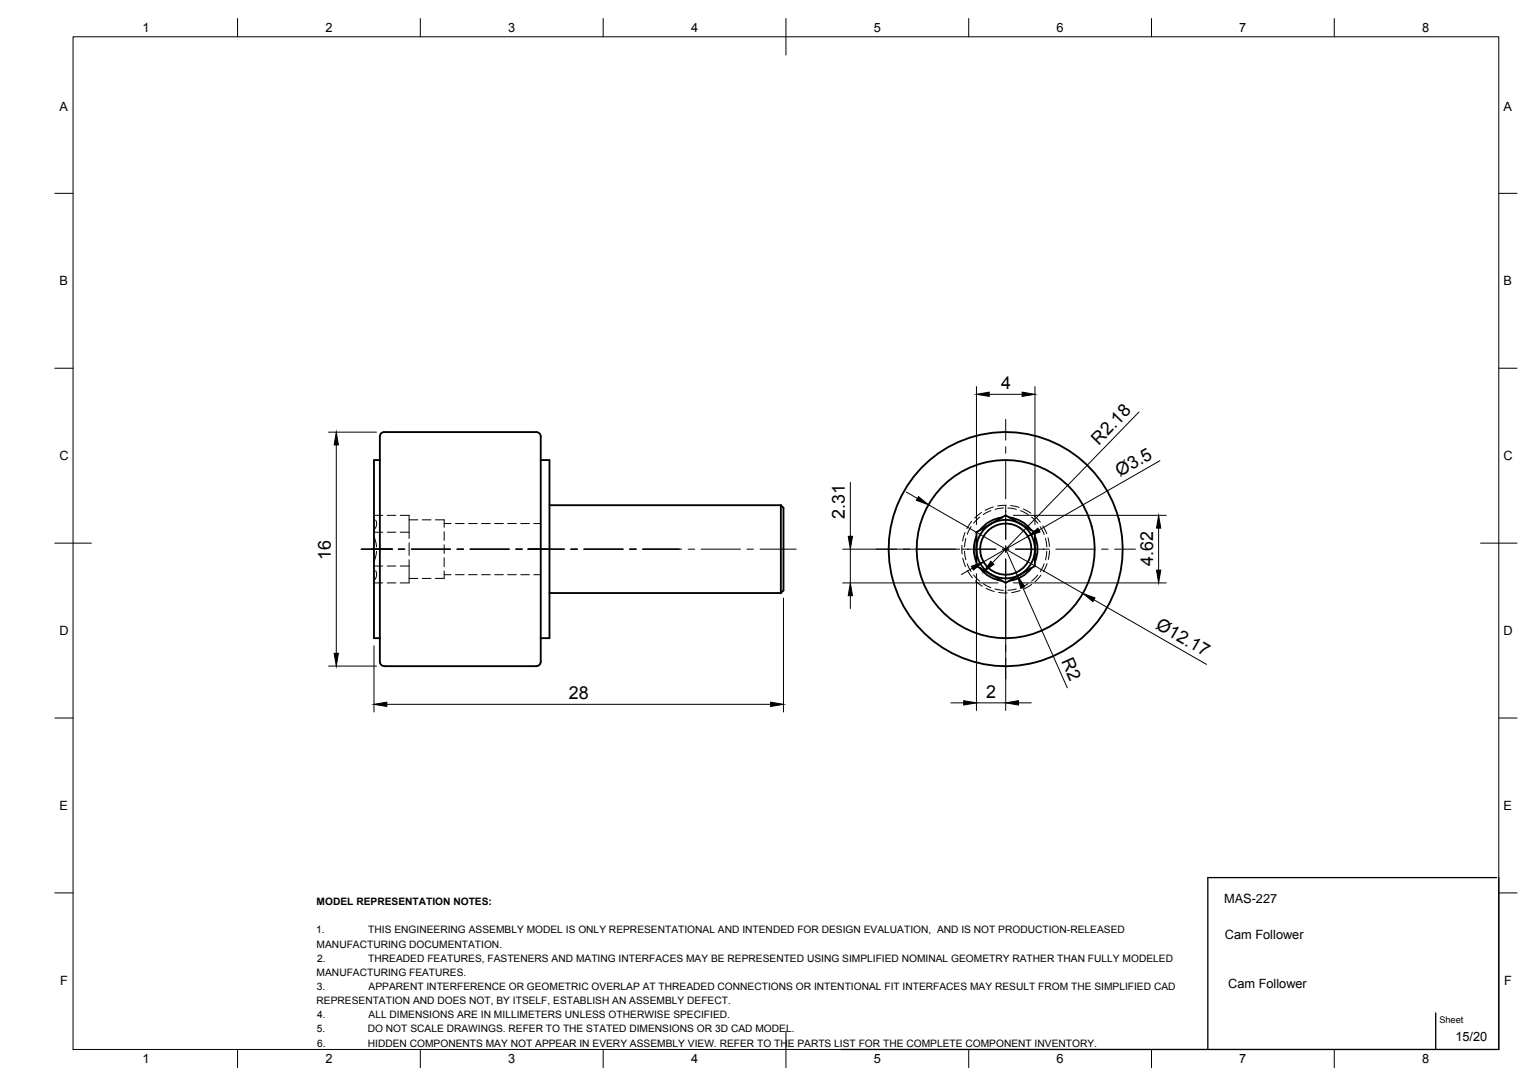
ISO-10303-21;
HEADER;
FILE_DESCRIPTION (('STEP AP214'),
    '1' );
FILE_NAME ( 'Cam Follower.step', '2026-10-06T08:24:41', ( '' ), ( '' ), 'STEP AP214', 'Unspecified', '' );
FILE_SCHEMA (( 'AUTOMOTIVE_DESIGN' ));
ENDSEC;
DATA;
#13=AXIS2_PLACEMENT_3D ( 'NONE', #19056, #4369, #12570 ) ;
#19=( CONVERSION_BASED_UNIT ( 'INCH', #19315 ) LENGTH_UNIT ( ) NAMED_UNIT ( #4330 ) ) ;
#26=AXIS2_PLACEMENT_3D ( 'NONE', #24045, #13033, #11185 ) ;
#76=ORIENTED_EDGE ( 'NONE', *, *, #16694, .F. ) ;
#94=DIRECTION ( 'NONE',  ( -1.000000000000000000, 0.000000000000000000, 0.000000000000000000 ) ) ;
#105=FILL_AREA_STYLE_COLOUR ( '', #1895 ) ;
#111=FACE_OUTER_BOUND ( 'NONE', #23572, .T. ) ;
#122=AXIS2_PLACEMENT_3D ( 'NONE', #22797, #14633, #3420 ) ;
#133=ORIENTED_EDGE ( 'NONE', *, *, #949, .F. ) ;
#142=ORIENTED_EDGE ( 'NONE', *, *, #15280, .T. ) ;
#147=VERTEX_POINT ( 'NONE', #612 ) ;
#148=CARTESIAN_POINT ( 'NONE',  ( 0.07874015748031495954, -0.04546065111729338803, -0.4724409448818898127 ) ) ;
#151=ORIENTED_EDGE ( 'NONE', *, *, #4349, .F. ) ;
#173=FACE_OUTER_BOUND ( 'NONE', #11804, .T. ) ;
#179=VECTOR ( 'NONE', #19878, 39.37007874015748143 ) ;
#197=CARTESIAN_POINT ( 'NONE',  ( -0.3149606299212598381, 0.000000000000000000, -0.03543307086614204404 ) ) ;
#217=CARTESIAN_POINT ( 'NONE',  ( -1.928513779527558736E-17, 0.000000000000000000, -0.4566929133858267376 ) ) ;
#241=EDGE_CURVE ( 'NONE', #21409, #11103, #22772, .T. ) ;
#262=DIRECTION ( 'NONE',  ( 0.8660254037844385966, 0.4999999999999998335, 0.000000000000000000 ) ) ;
#287=LINE ( 'NONE', #8993, #4640 ) ;
#289=ORIENTED_EDGE ( 'NONE', *, *, #13370, .F. ) ;
#294=ORIENTED_EDGE ( 'NONE', *, *, #2324, .F. ) ;
#295=VECTOR ( 'NONE', #17634, 39.37007874015748143 ) ;
#305=VECTOR ( 'NONE', #25355, 39.37007874015748854 ) ;
#307=ORIENTED_EDGE ( 'NONE', *, *, #13471, .F. ) ;
#340=CIRCLE ( 'NONE', #27828, 0.1181102362204724532 ) ;
#402=CYLINDRICAL_SURFACE ( 'NONE', #15048, 0.3149606299212598381 ) ;
#409=AXIS2_PLACEMENT_3D ( 'NONE', #960, #9547, #5473 ) ;
#417=DIRECTION ( 'NONE',  ( -0.000000000000000000, -0.000000000000000000, -1.000000000000000000 ) ) ;
#426=FACE_BOUND ( 'NONE', #2820, .T. ) ;
#444=DIRECTION ( 'NONE',  ( 0.000000000000000000, 0.000000000000000000, 1.000000000000000000 ) ) ;
#511=VECTOR ( 'NONE', #19555, 39.37007874015748143 ) ;
#534=ORIENTED_EDGE ( 'NONE', *, *, #21353, .T. ) ;
#572=CARTESIAN_POINT ( 'NONE',  ( 0.04957542349328453862, 0.06229891813554931657, -0.4653527282821430799 ) ) ;
#597=CARTESIAN_POINT ( 'NONE',  ( -1.928513779527558736E-17, 0.000000000000000000, -0.4448818897637791814 ) ) ;
#612=CARTESIAN_POINT ( 'NONE',  ( 0.07874015748238459567, -0.03414999754297557560, -0.4724409448841456749 ) ) ;
#617=EDGE_CURVE ( 'NONE', #8913, #147, #1095, .T. ) ;
#631=PLANE ( 'NONE',  #22046 ) ;
#638=DIRECTION ( 'NONE',  ( -1.000000000000000000, 0.000000000000000000, 0.000000000000000000 ) ) ;
#647=LINE ( 'NONE', #6869, #25949 ) ;
#681=CARTESIAN_POINT ( 'NONE',  ( 0.07874015748238459567, -0.03414999754297557560, -0.4724409448841456749 ) ) ;
#715=DIRECTION ( 'NONE',  ( 0.4999999999999998890, -0.8660254037844388186, 0.000000000000000000 ) ) ;
#771=AXIS2_PLACEMENT_3D ( 'NONE', #1458, #21348, #1986 ) ;
#785=ORIENTED_EDGE ( 'NONE', *, *, #9722, .F. ) ;
#791=FACE_OUTER_BOUND ( 'NONE', #25595, .T. ) ;
#797=CARTESIAN_POINT ( 'NONE',  ( -1.928513779527558736E-17, 0.000000000000000000, -0.03543307086614204404 ) ) ;
#841=ORIENTED_EDGE ( 'NONE', *, *, #19527, .T. ) ;
#851=AXIS2_PLACEMENT_3D ( 'NONE', #2037, #22857, #17156 ) ;
#859=PLANE ( 'NONE',  #25863 ) ;
#869=CARTESIAN_POINT ( 'NONE',  ( 0.06889763779527550980, 8.437527159479786693E-18, -0.2834645669291338543 ) ) ;
#876=DIRECTION ( 'NONE',  ( -0.8660254037844388186, 0.4999999999999998890, 0.000000000000000000 ) ) ;
#889=CIRCLE ( 'NONE', #13953, 0.08582677165167480748 ) ;
#895=FACE_OUTER_BOUND ( 'NONE', #5397, .T. ) ;
#922=ADVANCED_BREP_SHAPE_REPRESENTATION ( 'Cam Follower', ( #12666, #11588 ), #22004 ) ;
#926=SHAPE_DEFINITION_REPRESENTATION ( #15254, #6338 ) ;
#947=DIRECTION ( 'NONE',  ( 0.000000000000000000, 1.000000000000000000, 0.000000000000000000 ) ) ;
#949=EDGE_CURVE ( 'NONE', #26096, #20147, #2007, .T. ) ;
#960=CARTESIAN_POINT ( 'NONE',  ( -1.466875984251968630E-17, 0.000000000000000000, 0.000000000000000000 ) ) ;
#992=EDGE_CURVE ( 'NONE', #13219, #8587, #11932, .T. ) ;
#1028=DIRECTION ( 'NONE',  ( 0.000000000000000000, 0.000000000000000000, -1.000000000000000000 ) ) ;
#1072=AXIS2_PLACEMENT_3D ( 'NONE', #797, #26485, #22259 ) ;
#1076=ORIENTED_EDGE ( 'NONE', *, *, #5071, .F. ) ;
#1095=CIRCLE ( 'NONE', #20479, 0.08582677165167480748 ) ;
#1109=EDGE_CURVE ( 'NONE', #8913, #147, #3613, .T. ) ;
#1139=DIRECTION ( 'NONE',  ( 0.000000000000000000, 0.000000000000000000, 1.000000000000000000 ) ) ;
#1154=APPLICATION_CONTEXT ( 'automotive_design' ) ;
#1176=CARTESIAN_POINT ( 'NONE',  ( -0.009795313329799356164, 0.08526597544922019656, -0.4724409448841456749 ) ) ;
#1190=CARTESIAN_POINT ( 'NONE',  ( -0.08582677165167483524, 0.000000000000000000, -0.4724409448818898127 ) ) ;
#1215=ADVANCED_FACE ( 'NONE', ( #11828 ), #5648, .F. ) ;
#1220=LINE ( 'NONE', #9824, #25523 ) ;
#1227=DIRECTION ( 'NONE',  ( 1.000000000000000000, 0.000000000000000000, 0.000000000000000000 ) ) ;
#1268=DIRECTION ( 'NONE',  ( 0.000000000000000000, -1.000000000000000000, 0.000000000000000000 ) ) ;
#1279=DIRECTION ( 'NONE',  ( 1.000000000000000000, 0.000000000000000000, -0.000000000000000000 ) ) ;
#1309=DIRECTION ( 'NONE',  ( -1.000000000000000000, 0.000000000000000000, 0.000000000000000000 ) ) ;
#1314=AXIS2_PLACEMENT_3D ( 'NONE', #18114, #26761, #16038 ) ;
#1339=ORIENTED_EDGE ( 'NONE', *, *, #16589, .T. ) ;
#1349=CARTESIAN_POINT ( 'NONE',  ( 0.009795313329541911057, 0.08526597544697904485, -0.4724409448818898127 ) ) ;
#1370=DIRECTION ( 'NONE',  ( -0.000000000000000000, -0.000000000000000000, -1.000000000000000000 ) ) ;
#1407=ADVANCED_FACE ( 'NONE', ( #8707 ), #25945, .T. ) ;
#1444=EDGE_CURVE ( 'NONE', #22435, #24921, #647, .T. ) ;
#1458=CARTESIAN_POINT ( 'NONE',  ( -0.3031496062992123375, 0.000000000000000000, -0.03543307086614204404 ) ) ;
#1463=ORIENTED_EDGE ( 'NONE', *, *, #27662, .F. ) ;
#1464=CIRCLE ( 'NONE', #9132, 0.07874015748031489015 ) ;
#1465=DIRECTION ( 'NONE',  ( 0.000000000000000000, 0.000000000000000000, 1.000000000000000000 ) ) ;
#1467=AXIS2_PLACEMENT_3D ( 'NONE', #24695, #4934, #13548 ) ;
#1502=EDGE_CURVE ( 'NONE', #20698, #22435, #15499, .T. ) ;
#1510=FACE_OUTER_BOUND ( 'NONE', #14210, .T. ) ;
#1543=DIRECTION ( 'NONE',  ( 0.000000000000000000, 0.000000000000000000, -1.000000000000000000 ) ) ;
#1557=EDGE_LOOP ( 'NONE', ( #14465, #20326, #18276, #7986 ) ) ;
#1673=VERTEX_POINT ( 'NONE', #23799 ) ;
#1675=DIRECTION ( 'NONE',  ( -0.000000000000000000, -0.000000000000000000, -1.000000000000000000 ) ) ;
#1685=EDGE_CURVE ( 'NONE', #20128, #15627, #22080, .T. ) ;
#1708=EDGE_CURVE ( 'NONE', #2756, #15627, #3356, .T. ) ;
#1714=CIRCLE ( 'NONE', #26498, 0.2395669291338582696 ) ;
#1770=ORIENTED_EDGE ( 'NONE', *, *, #6491, .F. ) ;
#1867=VERTEX_POINT ( 'NONE', #26724 ) ;
#1873=CYLINDRICAL_SURFACE ( 'NONE', #17851, 0.2395669291338582696 ) ;
#1884=CARTESIAN_POINT ( 'NONE',  ( 0.07874015748031489015, 9.642888182262615344E-18, -0.3779527559055118058 ) ) ;
#1891=FACE_OUTER_BOUND ( 'NONE', #4069, .T. ) ;
#1895=COLOUR_RGB ( '', 0.40784314, 0.44705882, 0.49803922) ;
#1934=VERTEX_POINT ( 'NONE', #24403 ) ;
#1956=AXIS2_PLACEMENT_3D ( 'NONE', #9250, #22687, #14227 ) ;
#1962=ORIENTED_EDGE ( 'NONE', *, *, #1502, .T. ) ;
#1965=CARTESIAN_POINT ( 'NONE',  ( -1.928513779527558736E-17, 0.000000000000000000, -0.4566929133858267376 ) ) ;
#1986=DIRECTION ( 'NONE',  ( 0.000000000000000000, 0.000000000000000000, -1.000000000000000000 ) ) ;
#2007=CIRCLE ( 'NONE', #5137, 0.3149606299212598381 ) ;
#2037=CARTESIAN_POINT ( 'NONE',  ( 0.3031496062992122820, 3.712511950171106268E-17, -0.4448818897637791814 ) ) ;
#2066=EDGE_CURVE ( 'NONE', #2885, #6378, #9145, .T. ) ;
#2067=AXIS2_PLACEMENT_3D ( 'NONE', #10228, #4171, #8271 ) ;
#2129=ORIENTED_EDGE ( 'NONE', *, *, #13165, .F. ) ;
#2130=DIRECTION ( 'NONE',  ( 0.000000000000000000, 0.000000000000000000, -1.000000000000000000 ) ) ;
#2139=DIRECTION ( 'NONE',  ( -0.000000000000000000, -0.000000000000000000, -1.000000000000000000 ) ) ;
#2160=FACE_OUTER_BOUND ( 'NONE', #7511, .T. ) ;
#2171=CARTESIAN_POINT ( 'NONE',  ( 0.06894484415258525511, 0.05111597790624471116, -0.4724409448841456749 ) ) ;
#2198=LINE ( 'NONE', #2975, #8961 ) ;
#2218=ORIENTED_EDGE ( 'NONE', *, *, #241, .T. ) ;
#2227=ORIENTED_EDGE ( 'NONE', *, *, #22042, .F. ) ;
#2247=VERTEX_POINT ( 'NONE', #1349 ) ;
#2259=CARTESIAN_POINT ( 'NONE',  ( 0.000000000000000000, 0.000000000000000000, -0.4724409448818898127 ) ) ;
#2305=DIRECTION ( 'NONE',  ( -1.000000000000000000, 0.000000000000000000, 0.000000000000000000 ) ) ;
#2324=EDGE_CURVE ( 'NONE', #1867, #20809, #4761, .T. ) ;
#2360=EDGE_CURVE ( 'NONE', #24921, #21448, #25528, .T. ) ;
#2372=EDGE_CURVE ( 'NONE', #7271, #14162, #6429, .T. ) ;
#2381=ADVANCED_FACE ( 'NONE', ( #111 ), #4035, .F. ) ;
#2387=DIRECTION ( 'NONE',  ( 0.8660254037844382635, 0.5000000000000005551, 0.000000000000000000 ) ) ;
#2407=EDGE_LOOP ( 'NONE', ( #13278, #3298, #13573, #24116, #10984, #25647 ) ) ;
#2436=AXIS2_PLACEMENT_3D ( 'NONE', #217, #23645, #21376 ) ;
#2447=FILL_AREA_STYLE ('',( #105 ) ) ;
#2457=ORIENTED_EDGE ( 'NONE', *, *, #2066, .T. ) ;
#2463=FACE_OUTER_BOUND ( 'NONE', #1557, .T. ) ;
#2466=EDGE_CURVE ( 'NONE', #21409, #9119, #2876, .T. ) ;
#2467=PLANE ( 'NONE',  #7333 ) ;
#2492=DIRECTION ( 'NONE',  ( -1.000000000000000000, 0.000000000000000000, 0.000000000000000000 ) ) ;
#2513=LINE ( 'NONE', #7039, #22957 ) ;
#2525=CYLINDRICAL_SURFACE ( 'NONE', #25674, 0.1181102362204724532 ) ;
#2547=PLANE ( 'NONE',  #12830 ) ;
#2570=EDGE_CURVE ( 'NONE', #12477, #20698, #19211, .T. ) ;
#2582=LINE ( 'NONE', #17062, #18450 ) ;
#2590=DIRECTION ( 'NONE',  ( 1.000000000000000000, 0.000000000000000000, 0.000000000000000000 ) ) ;
#2632=AXIS2_PLACEMENT_3D ( 'NONE', #14783, #10215, #18829 ) ;
#2639=AXIS2_PLACEMENT_3D ( 'NONE', #27845, #16966, #4383 ) ;
#2650=CYLINDRICAL_SURFACE ( 'NONE', #4021, 0.3149606299212598381 ) ;
#2653=DIRECTION ( 'NONE',  ( -0.000000000000000000, -0.000000000000000000, -1.000000000000000000 ) ) ;
#2686=CIRCLE ( 'NONE', #13519, 0.07874015748031489015 ) ;
#2695=AXIS2_PLACEMENT_3D ( 'NONE', #25972, #417, #8999 ) ;
#2721=ORIENTED_EDGE ( 'NONE', *, *, #27018, .T. ) ;
#2732=DIRECTION ( 'NONE',  ( 0.000000000000000000, 0.000000000000000000, -1.000000000000000000 ) ) ;
#2744=CARTESIAN_POINT ( 'NONE',  ( 0.000000000000000000, 0.000000000000000000, -0.4724409448841456749 ) ) ;
#2756=VERTEX_POINT ( 'NONE', #6727 ) ;
#2768=EDGE_CURVE ( 'NONE', #7482, #18177, #8831, .T. ) ;
#2799=AXIS2_PLACEMENT_3D ( 'NONE', #20368, #22920, #1028 ) ;
#2820=EDGE_LOOP ( 'NONE', ( #12186, #18779 ) ) ;
#2876=B_SPLINE_CURVE_WITH_KNOTS ( 'NONE', 3,
 ( #15346, #23939, #8947, #6846, #15472, #15608 ),
 .UNSPECIFIED., .F., .F.,
 ( 4, 2, 4 ),
 ( 0.002631077521236949331, 0.003072896085239190580, 0.003514714649241431829 ),
 .UNSPECIFIED. ) ;
#2885=VERTEX_POINT ( 'NONE', #24357 ) ;
#2909=EDGE_CURVE ( 'NONE', #4618, #17370, #9814, .T. ) ;
#2928=ORIENTED_EDGE ( 'NONE', *, *, #27409, .F. ) ;
#2944=CARTESIAN_POINT ( 'NONE',  ( 0.01453548245982153216, 0.08252923752360777354, -0.4702630791244896136 ) ) ;
#2975=CARTESIAN_POINT ( 'NONE',  ( 0.06894484415506239861, -0.05111597790242464190, -0.4724409448818898127 ) ) ;
#2997=CARTESIAN_POINT ( 'NONE',  ( -0.06894484415077309358, 0.05111597790490104293, -0.4724409448818898127 ) ) ;
#3044=FACE_OUTER_BOUND ( 'NONE', #26076, .T. ) ;
#3065=AXIS2_PLACEMENT_3D ( 'NONE', #13857, #11454, #876 ) ;
#3066=ORIENTED_EDGE ( 'NONE', *, *, #5730, .T. ) ;
#3096=ORIENTED_EDGE ( 'NONE', *, *, #1444, .F. ) ;
#3114=ORIENTED_EDGE ( 'NONE', *, *, #27574, .T. ) ;
#3126=CARTESIAN_POINT ( 'NONE',  ( -4.821283464566928349E-18, 0.000000000000000000, -0.2834645669291338543 ) ) ;
#3238=DIRECTION ( 'NONE',  ( -0.000000000000000000, -0.000000000000000000, -1.000000000000000000 ) ) ;
#3242=CARTESIAN_POINT ( 'NONE',  ( -0.2395669291338582696, 0.000000000000000000, -0.4724409448818898127 ) ) ;
#3259=CARTESIAN_POINT ( 'NONE',  ( -0.06894484415077309358, 0.05111597790490104293, -0.4724409448818898127 ) ) ;
#3298=ORIENTED_EDGE ( 'NONE', *, *, #16372, .F. ) ;
#3301=FACE_OUTER_BOUND ( 'NONE', #4635, .T. ) ;
#3318=CARTESIAN_POINT ( 'NONE',  ( 0.2395669291338582696, 2.933848729453403498E-17, 0.000000000000000000 ) ) ;
#3329=EDGE_CURVE ( 'NONE', #8587, #13219, #1714, .T. ) ;
#3342=ORIENTED_EDGE ( 'NONE', *, *, #949, .T. ) ;
#3356=CIRCLE ( 'NONE', #21900, 0.07874015748031489015 ) ;
#3420=DIRECTION ( 'NONE',  ( -1.000000000000000000, 0.000000000000000000, 0.000000000000000000 ) ) ;
#3442=CARTESIAN_POINT ( 'NONE',  ( -0.07874015748031489015, 0.000000000000000000, -0.3779527559055118058 ) ) ;
#3527=CIRCLE ( 'NONE', #12131, 0.07874015748031489015 ) ;
#3542=VERTEX_POINT ( 'NONE', #27613 ) ;
#3573=ADVANCED_FACE ( 'NONE', ( #1891 ), #18981, .F. ) ;
#3579=VERTEX_POINT ( 'NONE', #17015 ) ;
#3597=ORIENTED_EDGE ( 'NONE', *, *, #10686, .F. ) ;
#3613=B_SPLINE_CURVE_WITH_KNOTS ( 'NONE', 3,
 ( #11138, #9009, #19895, #17630, #26250, #6910, #20029, #681 ),
 .UNSPECIFIED., .F., .F.,
 ( 4, 2, 2, 4 ),
 ( 0.001552469560294957029, 0.001994063167382608553, 0.002435656774470260078, 0.003318843988645562692 ),
 .UNSPECIFIED. ) ;
#3622=DIRECTION ( 'NONE',  ( 0.000000000000000000, 0.000000000000000000, -1.000000000000000000 ) ) ;
#3630=VERTEX_POINT ( 'NONE', #2171 ) ;
#3645=CARTESIAN_POINT ( 'NONE',  ( 0.000000000000000000, 0.000000000000000000, -0.4724409448841456749 ) ) ;
#3654=EDGE_CURVE ( 'NONE', #1673, #2756, #24054, .T. ) ;
#3665=DIRECTION ( 'NONE',  ( 0.000000000000000000, 0.000000000000000000, 1.000000000000000000 ) ) ;
#3684=PLANE ( 'NONE',  #4186 ) ;
#3699=ORIENTED_EDGE ( 'NONE', *, *, #19527, .F. ) ;
#3739=ORIENTED_EDGE ( 'NONE', *, *, #25748, .T. ) ;
#3769=AXIS2_PLACEMENT_3D ( 'NONE', #26947, #26798, #11404 ) ;
#3803=ADVANCED_FACE ( 'NONE', ( #1510 ), #25378, .F. ) ;
#3834=DIRECTION ( 'NONE',  ( -1.000000000000000000, -1.224646799147353454E-16, 0.000000000000000000 ) ) ;
#3868=VERTEX_POINT ( 'NONE', #7738 ) ;
#3871=CARTESIAN_POINT ( 'NONE',  ( -0.1110236220424516002, 0.000000000000000000, 0.6299212598425196763 ) ) ;
#3898=DIRECTION ( 'NONE',  ( 1.000000000000000000, 0.000000000000000000, 0.000000000000000000 ) ) ;
#3907=DIRECTION ( 'NONE',  ( 0.000000000000000000, 0.000000000000000000, 1.000000000000000000 ) ) ;
#3913=EDGE_LOOP ( 'NONE', ( #12682, #15515, #133, #1463 ) ) ;
#3963=DIRECTION ( 'NONE',  ( -0.000000000000000000, -0.000000000000000000, -1.000000000000000000 ) ) ;
#3986=CARTESIAN_POINT ( 'NONE',  ( 0.01928643301569668220, -0.07978627494126659669, -0.4680802598521938696 ) ) ;
#3995=EDGE_CURVE ( 'NONE', #26096, #10570, #24430, .T. ) ;
#4021=AXIS2_PLACEMENT_3D ( 'NONE', #24533, #11277, #15663 ) ;
#4035=PLANE ( 'NONE',  #25072 ) ;
#4061=VECTOR ( 'NONE', #262, 39.37007874015748854 ) ;
#4069=EDGE_LOOP ( 'NONE', ( #3739, #21924, #24634, #76, #3096, #7987, #5002 ) ) ;
#4091=CARTESIAN_POINT ( 'NONE',  ( 0.3031496062992122820, 3.784833611538078052E-17, -0.4566929133858267376 ) ) ;
#4123=EDGE_LOOP ( 'NONE', ( #4562, #26365 ) ) ;
#4170=EDGE_LOOP ( 'NONE', ( #7045, #1962, #27253 ) ) ;
#4171=DIRECTION ( 'NONE',  ( 0.000000000000000000, 0.000000000000000000, 1.000000000000000000 ) ) ;
#4172=CARTESIAN_POINT ( 'NONE',  ( 0.1110236220424516002, 1.359647233640338808E-17, 0.6299212598425196763 ) ) ;
#4186=AXIS2_PLACEMENT_3D ( 'NONE', #19375, #25313, #16985 ) ;
#4207=EDGE_LOOP ( 'NONE', ( #15106, #13124 ) ) ;
#4221=EDGE_LOOP ( 'NONE', ( #24244, #2218, #3066 ) ) ;
#4238=DIRECTION ( 'NONE',  ( -1.000000000000000000, 0.000000000000000000, 0.000000000000000000 ) ) ;
#4239=CARTESIAN_POINT ( 'NONE',  ( 0.000000000000000000, 0.000000000000000000, -0.4724409448818898127 ) ) ;
#4297=PRODUCT_DEFINITION_CONTEXT ( 'detailed design', #1154, 'design' ) ;
#4316=DIRECTION ( 'NONE',  ( 0.000000000000000000, 0.000000000000000000, -1.000000000000000000 ) ) ;
#4330=DIMENSIONAL_EXPONENTS ( 1.000000000000000000, 0.000000000000000000, 0.000000000000000000, 0.000000000000000000, 0.000000000000000000, 0.000000000000000000, 0.000000000000000000 ) ;
#4346=ORIENTED_EDGE ( 'NONE', *, *, #2909, .T. ) ;
#4349=EDGE_CURVE ( 'NONE', #7482, #3868, #8097, .T. ) ;
#4353=TOROIDAL_SURFACE ( 'NONE', #21954, 0.3031496062992122820, 0.01181102362204755792 ) ;
#4369=DIRECTION ( 'NONE',  ( 0.000000000000000000, 0.000000000000000000, -1.000000000000000000 ) ) ;
#4383=DIRECTION ( 'NONE',  ( -1.000000000000000000, 0.000000000000000000, 0.000000000000000000 ) ) ;
#4493=DIRECTION ( 'NONE',  ( -0.000000000000000000, -0.000000000000000000, -1.000000000000000000 ) ) ;
#4506=EDGE_CURVE ( 'NONE', #12477, #26781, #2582, .T. ) ;
#4562=ORIENTED_EDGE ( 'NONE', *, *, #2324, .T. ) ;
#4611=VECTOR ( 'NONE', #3907, 39.37007874015748143 ) ;
#4614=FACE_OUTER_BOUND ( 'NONE', #15635, .T. ) ;
#4618=VERTEX_POINT ( 'NONE', #22357 ) ;
#4623=CARTESIAN_POINT ( 'NONE',  ( -0.07874015748031495954, -0.04546065111729338803, -0.4724409448818898127 ) ) ;
#4635=EDGE_LOOP ( 'NONE', ( #142, #12752 ) ) ;
#4640=VECTOR ( 'NONE', #11392, 39.37007874015748143 ) ;
#4679=EDGE_CURVE ( 'NONE', #14162, #3630, #27583, .T. ) ;
#4687=CARTESIAN_POINT ( 'NONE',  ( 0.000000000000000000, 0.000000000000000000, -0.4724409448841456749 ) ) ;
#4690=DIRECTION ( 'NONE',  ( -0.8660254037844382635, -0.5000000000000005551, 0.000000000000000000 ) ) ;
#4727=EDGE_LOOP ( 'NONE', ( #14075, #24927 ) ) ;
#4742=LINE ( 'NONE', #148, #10499 ) ;
#4761=CIRCLE ( 'NONE', #2067, 0.1110236220424516002 ) ;
#4767=FACE_OUTER_BOUND ( 'NONE', #8375, .T. ) ;
#4805=VERTEX_POINT ( 'NONE', #21773 ) ;
#4825=CARTESIAN_POINT ( 'NONE',  ( 0.07874015748031495954, 0.04546065111729338803, -0.3779527559055118058 ) ) ;
#4834=FACE_BOUND ( 'NONE', #5849, .T. ) ;
#4835=ADVANCED_FACE ( 'NONE', ( #3044 ), #5041, .T. ) ;
#4860=CARTESIAN_POINT ( 'NONE',  ( -1.466875984251968630E-17, 0.000000000000000000, -0.4724409448818898127 ) ) ;
#4884=FACE_OUTER_BOUND ( 'NONE', #19252, .T. ) ;
#4934=DIRECTION ( 'NONE',  ( 0.000000000000000000, 0.000000000000000000, -1.000000000000000000 ) ) ;
#4935=ORIENTED_EDGE ( 'NONE', *, *, #25296, .T. ) ;
#4949=ORIENTED_EDGE ( 'NONE', *, *, #11130, .F. ) ;
#4950=DIRECTION ( 'NONE',  ( 0.000000000000000000, -1.000000000000000000, 0.000000000000000000 ) ) ;
#4962=DIRECTION ( 'NONE',  ( -1.000000000000000000, 0.000000000000000000, 0.000000000000000000 ) ) ;
#4991=DIRECTION ( 'NONE',  ( 0.000000000000000000, -1.000000000000000000, 0.000000000000000000 ) ) ;
#5002=ORIENTED_EDGE ( 'NONE', *, *, #16148, .F. ) ;
#5010=DIRECTION ( 'NONE',  ( -1.000000000000000000, 0.000000000000000000, 0.000000000000000000 ) ) ;
#5041=CYLINDRICAL_SURFACE ( 'NONE', #409, 0.2395669291338582696 ) ;
#5045=CARTESIAN_POINT ( 'NONE',  ( -0.05945372446461825305, -0.05659567841061365762, -0.4680802598521939806 ) ) ;
#5054=FACE_OUTER_BOUND ( 'NONE', #11043, .T. ) ;
#5071=EDGE_CURVE ( 'NONE', #26781, #27801, #26866, .T. ) ;
#5080=DIRECTION ( 'NONE',  ( 0.000000000000000000, 0.000000000000000000, -1.000000000000000000 ) ) ;
#5083=ORIENTED_EDGE ( 'NONE', *, *, #19523, .F. ) ;
#5089=ORIENTED_EDGE ( 'NONE', *, *, #18442, .T. ) ;
#5121=CARTESIAN_POINT ( 'NONE',  ( -1.466875984251968630E-17, 0.000000000000000000, -0.02362204724409448786 ) ) ;
#5123=DIRECTION ( 'NONE',  ( -1.000000000000000000, 0.000000000000000000, 0.000000000000000000 ) ) ;
#5124=ORIENTED_EDGE ( 'NONE', *, *, #22846, .T. ) ;
#5125=AXIS2_PLACEMENT_3D ( 'NONE', #13732, #11340, #15599 ) ;
#5130=VECTOR ( 'NONE', #4991, 39.37007874015748143 ) ;
#5137=AXIS2_PLACEMENT_3D ( 'NONE', #27832, #8468, #4238 ) ;
#5183=CARTESIAN_POINT ( 'NONE',  ( -0.009795313329541911057, -0.08526597544697904485, -0.4724409448818898127 ) ) ;
#5212=CARTESIAN_POINT ( 'NONE',  ( 0.2395669291338582696, 2.933848729453403498E-17, -0.4566929133858267376 ) ) ;
#5213=CARTESIAN_POINT ( 'NONE',  ( 0.05945372446461825305, 0.05659567841061365762, -0.4680802598521939806 ) ) ;
#5229=CARTESIAN_POINT ( 'NONE',  ( 0.000000000000000000, 0.000000000000000000, 0.000000000000000000 ) ) ;
#5267=VERTEX_POINT ( 'NONE', #9743 ) ;
#5273=ORIENTED_EDGE ( 'NONE', *, *, #11599, .T. ) ;
#5294=VECTOR ( 'NONE', #1675, 39.37007874015748143 ) ;
#5312=VERTEX_POINT ( 'NONE', #23330 ) ;
#5315=LINE ( 'NONE', #20291, #27238 ) ;
#5357=ADVANCED_FACE ( 'NONE', ( #4767 ), #2650, .T. ) ;
#5361=LINE ( 'NONE', #5212, #18750 ) ;
#5363=CIRCLE ( 'NONE', #851, 0.01181102362204754924 ) ;
#5397=EDGE_LOOP ( 'NONE', ( #10780, #27110 ) ) ;
#5424=EDGE_CURVE ( 'NONE', #20128, #6015, #2513, .T. ) ;
#5430=ORIENTED_EDGE ( 'NONE', *, *, #2909, .F. ) ;
#5441=UNCERTAINTY_MEASURE_WITH_UNIT (LENGTH_MEASURE( 1.000000000000000082E-05 ), #19, 'distance_accuracy_value', 'NONE') ;
#5472=EDGE_CURVE ( 'NONE', #10266, #9518, #21080, .T. ) ;
#5473=DIRECTION ( 'NONE',  ( -1.000000000000000000, 0.000000000000000000, 0.000000000000000000 ) ) ;
#5499=MECHANICAL_DESIGN_GEOMETRIC_PRESENTATION_REPRESENTATION('',(#27617),#17674);
#5507=DIRECTION ( 'NONE',  ( -1.000000000000000000, 0.000000000000000000, 0.000000000000000000 ) ) ;
#5517=CARTESIAN_POINT ( 'NONE',  ( -9.160727710493059047E-17, 0.000000000000000000, -0.02362204724409468909 ) ) ;
#5543=CARTESIAN_POINT ( 'NONE',  ( -0.08582677165393072516, 0.000000000000000000, -0.4724409448841456749 ) ) ;
#5552=EDGE_CURVE ( 'NONE', #23745, #23749, #5363, .T. ) ;
#5586=ADVANCED_FACE ( 'NONE', ( #18590 ), #13959, .T. ) ;
#5589=LINE ( 'NONE', #3442, #7088 ) ;
#5615=ORIENTED_EDGE ( 'NONE', *, *, #7592, .T. ) ;
#5635=VERTEX_POINT ( 'NONE', #7883 ) ;
#5648=CONICAL_SURFACE ( 'NONE', #25034, 0.08582677165393072516, 0.7853981625000011624 ) ;
#5661=ORIENTED_EDGE ( 'NONE', *, *, #13984, .T. ) ;
#5689=AXIS2_PLACEMENT_3D ( 'NONE', #21404, #8545, #17163 ) ;
#5730=EDGE_CURVE ( 'NONE', #11103, #9119, #22977, .T. ) ;
#5738=ADVANCED_FACE ( 'NONE', ( #8467 ), #22051, .F. ) ;
#5770=DIRECTION ( 'NONE',  ( 0.000000000000000000, 0.000000000000000000, -1.000000000000000000 ) ) ;
#5834=CARTESIAN_POINT ( 'NONE',  ( 0.04448665381632212201, -0.06523692067838748887, -0.4653551329966303385 ) ) ;
#5849=EDGE_LOOP ( 'NONE', ( #7073, #17608 ) ) ;
#5881=EDGE_CURVE ( 'NONE', #2885, #8441, #18904, .T. ) ;
#5915=ORIENTED_EDGE ( 'NONE', *, *, #27409, .T. ) ;
#6015=VERTEX_POINT ( 'NONE', #17564 ) ;
#6024=AXIS2_PLACEMENT_3D ( 'NONE', #19196, #23324, #18909 ) ;
#6030=EDGE_LOOP ( 'NONE', ( #3114, #9421 ) ) ;
#6058=ORIENTED_EDGE ( 'NONE', *, *, #7177, .T. ) ;
#6116=ORIENTED_EDGE ( 'NONE', *, *, #617, .T. ) ;
#6120=CARTESIAN_POINT ( 'NONE',  ( 0.06894484415077314909, -0.05111597790490109150, -0.4724409448818898127 ) ) ;
#6135=DIRECTION ( 'NONE',  ( -1.000000000000000000, 0.000000000000000000, 0.000000000000000000 ) ) ;
#6161=ORIENTED_EDGE ( 'NONE', *, *, #1708, .F. ) ;
#6174=ORIENTED_EDGE ( 'NONE', *, *, #23058, .F. ) ;
#6194=CARTESIAN_POINT ( 'NONE',  ( 0.000000000000000000, 0.000000000000000000, -0.3779527559055118058 ) ) ;
#6252=CARTESIAN_POINT ( 'NONE',  ( -4.821283464566928349E-18, 0.000000000000000000, -0.3779527559055118058 ) ) ;
#6277=LINE ( 'NONE', #3871, #10048 ) ;
#6285=VECTOR ( 'NONE', #11721, 39.37007874015748143 ) ;
#6302=AXIS2_PLACEMENT_3D ( 'NONE', #12976, #17365, #8604 ) ;
#6308=ORIENTED_EDGE ( 'NONE', *, *, #23058, .T. ) ;
#6338=SHAPE_REPRESENTATION ( 'Cam Follower', ( #11588 ), #22004 ) ;
#6340=ADVANCED_FACE ( 'NONE', ( #11819 ), #20435, .F. ) ;
#6378=VERTEX_POINT ( 'NONE', #16763 ) ;
#6429=LINE ( 'NONE', #18844, #27794 ) ;
#6467=CARTESIAN_POINT ( 'NONE',  ( 0.000000000000000000, 0.000000000000000000, 0.6299212598425196763 ) ) ;
#6475=CARTESIAN_POINT ( 'NONE',  ( -1.928513779527558736E-17, 0.000000000000000000, -0.4448818897637791814 ) ) ;
#6488=CARTESIAN_POINT ( 'NONE',  ( -0.07874015748031495954, -1.062017969535966354E-23, -0.4653543306978102367 ) ) ;
#6491=EDGE_CURVE ( 'NONE', #6015, #5312, #26470, .T. ) ;
#6500=LINE ( 'NONE', #27562, #14787 ) ;
#6532=ORIENTED_EDGE ( 'NONE', *, *, #24900, .T. ) ;
#6566=SURFACE_STYLE_FILL_AREA ( #2447 ) ;
#6635=CARTESIAN_POINT ( 'NONE',  ( 0.07874015748031495954, 0.04546065111729338803, -0.4724409448818898127 ) ) ;
#6672=ORIENTED_EDGE ( 'NONE', *, *, #14295, .T. ) ;
#6678=CARTESIAN_POINT ( 'NONE',  ( 0.000000000000000000, -0.09092130223458683158, -0.3779527559055118058 ) ) ;
#6723=AXIS2_PLACEMENT_3D ( 'NONE', #14094, #5770, #14250 ) ;
#6724=CARTESIAN_POINT ( 'NONE',  ( 0.000000000000000000, 0.000000000000000000, -0.4724409448818898127 ) ) ;
#6727=CARTESIAN_POINT ( 'NONE',  ( 0.03937007874015749365, -0.06819097667593998491, -0.3779527559055118058 ) ) ;
#6766=AXIS2_PLACEMENT_3D ( 'NONE', #7584, #14084, #22698 ) ;
#6829=ORIENTED_EDGE ( 'NONE', *, *, #20642, .T. ) ;
#6841=CARTESIAN_POINT ( 'NONE',  ( 0.000000000000000000, -0.09092130223458683158, -0.3779527559055118058 ) ) ;
#6846=CARTESIAN_POINT ( 'NONE',  ( -0.07874015748031495954, 0.02307066120096010892, -0.4684762439721033012 ) ) ;
#6869=CARTESIAN_POINT ( 'NONE',  ( 0.000000000000000000, 0.09092130223458683158, -0.3779527559055118058 ) ) ;
#6871=CARTESIAN_POINT ( 'NONE',  ( -0.03937007874015754916, -0.06819097667594005430, -0.3779527559055118058 ) ) ;
#6876=EDGE_LOOP ( 'NONE', ( #6058, #6672 ) ) ;
#6877=AXIS2_PLACEMENT_3D ( 'NONE', #16800, #7907, #20474 ) ;
#6909=CARTESIAN_POINT ( 'NONE',  ( -0.06894484415258525511, -0.05111597790624471116, -0.4724409448841456749 ) ) ;
#6910=CARTESIAN_POINT ( 'NONE',  ( 0.07874015748031498729, -0.01181388133159171419, -0.4653549736499515421 ) ) ;
#6941=CARTESIAN_POINT ( 'NONE',  ( 0.000000000000000000, 0.000000000000000000, 0.6299212598425196763 ) ) ;
#6984=AXIS2_PLACEMENT_3D ( 'NONE', #26690, #22465, #18627 ) ;
#7026=ORIENTED_EDGE ( 'NONE', *, *, #16884, .T. ) ;
#7039=CARTESIAN_POINT ( 'NONE',  ( 0.000000000000000000, -0.09092130223458683158, -0.3779527559055118058 ) ) ;
#7042=CARTESIAN_POINT ( 'NONE',  ( 0.06889763779527550980, 0.000000000000000000, -0.2834645669291338543 ) ) ;
#7045=ORIENTED_EDGE ( 'NONE', *, *, #18252, .F. ) ;
#7047=VERTEX_POINT ( 'NONE', #23024 ) ;
#7073=ORIENTED_EDGE ( 'NONE', *, *, #18790, .F. ) ;
#7088=VECTOR ( 'NONE', #12358, 39.37007874015748143 ) ;
#7136=VECTOR ( 'NONE', #4690, 39.37007874015748854 ) ;
#7156=CARTESIAN_POINT ( 'NONE',  ( 0.000000000000000000, 0.000000000000000000, 0.6228346456772185791 ) ) ;
#7177=EDGE_CURVE ( 'NONE', #7047, #16467, #13998, .T. ) ;
#7202=CARTESIAN_POINT ( 'NONE',  ( 0.009795313329541911057, 0.08526597544697904485, -0.4724409448818898127 ) ) ;
#7208=FACE_OUTER_BOUND ( 'NONE', #8008, .T. ) ;
#7271=VERTEX_POINT ( 'NONE', #10709 ) ;
#7330=AXIS2_PLACEMENT_3D ( 'NONE', #5121, #26881, #16297 ) ;
#7333=AXIS2_PLACEMENT_3D ( 'NONE', #6724, #2732, #26199 ) ;
#7360=ORIENTED_EDGE ( 'NONE', *, *, #1708, .T. ) ;
#7361=ORIENTED_EDGE ( 'NONE', *, *, #22319, .T. ) ;
#7477=DIRECTION ( 'NONE',  ( 0.000000000000000000, 0.000000000000000000, -1.000000000000000000 ) ) ;
#7482=VERTEX_POINT ( 'NONE', #3318 ) ;
#7503=ORIENTED_EDGE ( 'NONE', *, *, #18790, .T. ) ;
#7511=EDGE_LOOP ( 'NONE', ( #6161, #22048, #13340 ) ) ;
#7574=CARTESIAN_POINT ( 'NONE',  ( -1.928513779527558736E-17, 0.000000000000000000, -0.02362204724409448786 ) ) ;
#7580=DIRECTION ( 'NONE',  ( -1.000000000000000000, 0.000000000000000000, 0.000000000000000000 ) ) ;
#7584=CARTESIAN_POINT ( 'NONE',  ( -4.821283464566928349E-18, 0.000000000000000000, -0.3779527559055118058 ) ) ;
#7592=EDGE_CURVE ( 'NONE', #23745, #10570, #24386, .T. ) ;
#7644=CARTESIAN_POINT ( 'NONE',  ( -0.07874015748031495954, 0.04546065111729338803, -0.3779527559055118058 ) ) ;
#7717=DIRECTION ( 'NONE',  ( 0.8660254037844385966, -0.4999999999999998335, 0.000000000000000000 ) ) ;
#7738=CARTESIAN_POINT ( 'NONE',  ( -0.2395669291338582696, 0.000000000000000000, 0.000000000000000000 ) ) ;
#7780=FACE_OUTER_BOUND ( 'NONE', #6876, .T. ) ;
#7845=CIRCLE ( 'NONE', #8743, 0.3031496062992122820 ) ;
#7882=ORIENTED_EDGE ( 'NONE', *, *, #12632, .F. ) ;
#7883=CARTESIAN_POINT ( 'NONE',  ( 0.000000000000000000, 0.09092130223458683158, -0.4724409448818898127 ) ) ;
#7897=AXIS2_PLACEMENT_3D ( 'NONE', #4239, #10442, #8342 ) ;
#7907=DIRECTION ( 'NONE',  ( 0.000000000000000000, 0.000000000000000000, -1.000000000000000000 ) ) ;
#7923=DIRECTION ( 'NONE',  ( 1.000000000000000000, 0.000000000000000000, 0.000000000000000000 ) ) ;
#7985=ORIENTED_EDGE ( 'NONE', *, *, #20054, .F. ) ;
#7986=ORIENTED_EDGE ( 'NONE', *, *, #20028, .F. ) ;
#7987=ORIENTED_EDGE ( 'NONE', *, *, #12632, .T. ) ;
#8008=EDGE_LOOP ( 'NONE', ( #5661, #14370 ) ) ;
#8092=EDGE_LOOP ( 'NONE', ( #10502, #13646, #17576, #1076, #16394, #6174, #7026, #14818 ) ) ;
#8097=CIRCLE ( 'NONE', #11186, 0.2395669291338582696 ) ;
#8102=CARTESIAN_POINT ( 'NONE',  ( 0.000000000000000000, 0.09092130223458683158, -0.4724409448818898127 ) ) ;
#8105=DIRECTION ( 'NONE',  ( 1.000000000000000000, 0.000000000000000000, 0.000000000000000000 ) ) ;
#8150=ADVANCED_FACE ( 'NONE', ( #19776 ), #12758, .T. ) ;
#8163=CIRCLE ( 'NONE', #23504, 0.1181102362204724532 ) ;
#8174=SHAPE_REPRESENTATION_RELATIONSHIP ( 'NONE' , 'NONE' ,  #6338, #922 ) ;
#8179=ORIENTED_EDGE ( 'NONE', *, *, #2570, .F. ) ;
#8220=VERTEX_POINT ( 'NONE', #9641 ) ;
#8232=AXIS2_PLACEMENT_3D ( 'NONE', #13199, #21829, #19708 ) ;
#8252=VECTOR ( 'NONE', #10782, 39.37007874015748143 ) ;
#8271=DIRECTION ( 'NONE',  ( 1.000000000000000000, 0.000000000000000000, 0.000000000000000000 ) ) ;
#8285=LINE ( 'NONE', #13070, #13513 ) ;
#8342=DIRECTION ( 'NONE',  ( -1.000000000000000000, 0.000000000000000000, 0.000000000000000000 ) ) ;
#8349=CARTESIAN_POINT ( 'NONE',  ( 0.000000000000000000, 0.09092130223458683158, -0.3779527559055118058 ) ) ;
#8371=FACE_OUTER_BOUND ( 'NONE', #10504, .T. ) ;
#8375=EDGE_LOOP ( 'NONE', ( #3342, #15180, #5615, #14706 ) ) ;
#8377=EDGE_CURVE ( 'NONE', #17187, #21448, #16721, .T. ) ;
#8383=CARTESIAN_POINT ( 'NONE',  ( -1.466875984251968630E-17, 0.000000000000000000, -0.4566929133858267376 ) ) ;
#8428=CARTESIAN_POINT ( 'NONE',  ( 0.07874015748031495954, -0.04546065111729338803, -0.4724409448818898127 ) ) ;
#8440=ORIENTED_EDGE ( 'NONE', *, *, #11042, .T. ) ;
#8441=VERTEX_POINT ( 'NONE', #10205 ) ;
#8467=FACE_OUTER_BOUND ( 'NONE', #4221, .T. ) ;
#8468=DIRECTION ( 'NONE',  ( 0.000000000000000000, 0.000000000000000000, -1.000000000000000000 ) ) ;
#8523=CARTESIAN_POINT ( 'NONE',  ( 0.000000000000000000, 0.000000000000000000, 0.6299212598425196763 ) ) ;
#8524=EDGE_CURVE ( 'NONE', #2247, #3630, #19934, .T. ) ;
#8541=CARTESIAN_POINT ( 'NONE',  ( 0.000000000000000000, 0.09092130223458683158, -0.3779527559055118058 ) ) ;
#8545=DIRECTION ( 'NONE',  ( -0.000000000000000000, -0.000000000000000000, -1.000000000000000000 ) ) ;
#8562=DIRECTION ( 'NONE',  ( 0.8660254037844385966, 0.4999999999999998335, 0.000000000000000000 ) ) ;
#8587=VERTEX_POINT ( 'NONE', #10779 ) ;
#8604=DIRECTION ( 'NONE',  ( -1.000000000000000000, 0.000000000000000000, 0.000000000000000000 ) ) ;
#8616=B_SPLINE_CURVE_WITH_KNOTS ( 'NONE', 3,
 ( #6120, #14755, #14604, #21068, #5834, #12601, #3986, #23361 ),
 .UNSPECIFIED., .F., .F.,
 ( 4, 2, 2, 4 ),
 ( 5.336250286676794493E-07, 0.0004434172983717934590, 0.0008863009717149191629, 0.001772068318401170788 ),
 .UNSPECIFIED. ) ;
#8679=DIRECTION ( 'NONE',  ( 0.000000000000000000, 0.000000000000000000, -1.000000000000000000 ) ) ;
#8683=ADVANCED_FACE ( 'NONE', ( #25302 ), #23055, .T. ) ;
#8690=LINE ( 'NONE', #15618, #18327 ) ;
#8707=FACE_OUTER_BOUND ( 'NONE', #27744, .T. ) ;
#8719=CYLINDRICAL_SURFACE ( 'NONE', #25858, 0.1181102362204724532 ) ;
#8732=VECTOR ( 'NONE', #11467, 39.37007874015748143 ) ;
#8743=AXIS2_PLACEMENT_3D ( 'NONE', #7574, #11958, #20577 ) ;
#8754=VECTOR ( 'NONE', #25803, 39.37007874015748143 ) ;
#8788=CIRCLE ( 'NONE', #10602, 0.2395669291338582696 ) ;
#8790=CIRCLE ( 'NONE', #16916, 0.3031496062992122820 ) ;
#8813=( NAMED_UNIT ( * ) SI_UNIT ( $, .STERADIAN. ) SOLID_ANGLE_UNIT ( ) ) ;
#8831=LINE ( 'NONE', #19293, #5294 ) ;
#8835=ORIENTED_EDGE ( 'NONE', *, *, #24370, .T. ) ;
#8895=DIRECTION ( 'NONE',  ( 0.000000000000000000, 1.000000000000000000, 0.000000000000000000 ) ) ;
#8909=AXIS2_PLACEMENT_3D ( 'NONE', #4860, #9661, #638 ) ;
#8913=VERTEX_POINT ( 'NONE', #19651 ) ;
#8915=ORIENTED_EDGE ( 'NONE', *, *, #15075, .T. ) ;
#8940=VECTOR ( 'NONE', #18515, 39.37007874015748143 ) ;
#8946=EDGE_CURVE ( 'NONE', #6378, #8220, #16334, .T. ) ;
#8947=CARTESIAN_POINT ( 'NONE',  ( -0.07874015748031495954, 0.01169115616675828022, -0.4660234066338417858 ) ) ;
#8961=VECTOR ( 'NONE', #8562, 39.37007874015748854 ) ;
#8993=CARTESIAN_POINT ( 'NONE',  ( -0.1181102362204724532, 0.000000000000000000, 0.6299212598425196763 ) ) ;
#8999=DIRECTION ( 'NONE',  ( -1.000000000000000000, 0.000000000000000000, 0.000000000000000000 ) ) ;
#9009=CARTESIAN_POINT ( 'NONE',  ( 0.07874015748031495954, 0.02870816175736372669, -0.4702756685301184292 ) ) ;
#9010=CARTESIAN_POINT ( 'NONE',  ( -4.821283464566928349E-18, 0.000000000000000000, -0.3779527559055118058 ) ) ;
#9018=VECTOR ( 'NONE', #26167, 39.37007874015748854 ) ;
#9020=CARTESIAN_POINT ( 'NONE',  ( -0.009795313329799356164, 0.08526597544922019656, -0.4724409448841456749 ) ) ;
#9056=APPLICATION_CONTEXT ( 'automotive_design' ) ;
#9090=DIRECTION ( 'NONE',  ( -1.000000000000000000, 0.000000000000000000, -0.000000000000000000 ) ) ;
#9119=VERTEX_POINT ( 'NONE', #24158 ) ;
#9127=ADVANCED_FACE ( 'NONE', ( #13689 ), #16355, .T. ) ;
#9132=AXIS2_PLACEMENT_3D ( 'NONE', #11912, #18387, #22509 ) ;
#9145=LINE ( 'NONE', #15666, #295 ) ;
#9151=EDGE_LOOP ( 'NONE', ( #9394, #21259, #4346, #2928 ) ) ;
#9156=CARTESIAN_POINT ( 'NONE',  ( 0.3149606299212598381, 3.857155272905049219E-17, -0.03543307086614173179 ) ) ;
#9167=ADVANCED_FACE ( 'NONE', ( #11299 ), #15898, .F. ) ;
#9189=B_SPLINE_CURVE_WITH_KNOTS ( 'NONE', 3,
 ( #3259, #16002, #24889, #20519, #16147, #10053, #24745, #1176 ),
 .UNSPECIFIED., .F., .F.,
 ( 4, 2, 2, 4 ),
 ( 5.336250286684417789E-07, 0.0004434172983717937842, 0.0008863009717149190544, 0.001772068318401169270 ),
 .UNSPECIFIED. ) ;
#9195=ADVANCED_FACE ( 'NONE', ( #25127 ), #24847, .F. ) ;
#9203=PLANE ( 'NONE',  #5125 ) ;
#9217=DIRECTION ( 'NONE',  ( 0.000000000000000000, 0.000000000000000000, 1.000000000000000000 ) ) ;
#9218=ORIENTED_EDGE ( 'NONE', *, *, #5424, .T. ) ;
#9228=ADVANCED_FACE ( 'NONE', ( #14417 ), #18473, .T. ) ;
#9235=ORIENTED_EDGE ( 'NONE', *, *, #18442, .F. ) ;
#9242=CARTESIAN_POINT ( 'NONE',  ( -1.928513779527558736E-17, 0.000000000000000000, -0.03543307086614173179 ) ) ;
#9250=CARTESIAN_POINT ( 'NONE',  ( 0.000000000000000000, 0.000000000000000000, 0.6299212598425196763 ) ) ;
#9273=VECTOR ( 'NONE', #22934, 39.37007874015748143 ) ;
#9288=EDGE_CURVE ( 'NONE', #7271, #21448, #11999, .T. ) ;
#9305=DIRECTION ( 'NONE',  ( 0.000000000000000000, 0.000000000000000000, -1.000000000000000000 ) ) ;
#9327=ORIENTED_EDGE ( 'NONE', *, *, #6491, .T. ) ;
#9332=ADVANCED_FACE ( 'NONE', ( #13344, #17586 ), #2467, .T. ) ;
#9384=CARTESIAN_POINT ( 'NONE',  ( 0.000000000000000000, -0.09092130223458683158, -0.3779527559055118058 ) ) ;
#9394=ORIENTED_EDGE ( 'NONE', *, *, #992, .F. ) ;
#9421=ORIENTED_EDGE ( 'NONE', *, *, #5472, .F. ) ;
#9501=CARTESIAN_POINT ( 'NONE',  ( -0.07874015748031495954, 0.04546065111729338803, -0.4724409448818898127 ) ) ;
#9518=VERTEX_POINT ( 'NONE', #21389 ) ;
#9536=EDGE_LOOP ( 'NONE', ( #23774, #17213, #27563 ) ) ;
#9547=DIRECTION ( 'NONE',  ( -0.000000000000000000, -0.000000000000000000, -1.000000000000000000 ) ) ;
#9554=CARTESIAN_POINT ( 'NONE',  ( -0.01453548245982153216, -0.08252923752360777354, -0.4702630791244896136 ) ) ;
#9608=EDGE_CURVE ( 'NONE', #1867, #8441, #6277, .T. ) ;
#9641=CARTESIAN_POINT ( 'NONE',  ( -0.1181102362204724532, 0.000000000000000000, 0.000000000000000000 ) ) ;
#9661=DIRECTION ( 'NONE',  ( 0.000000000000000000, 0.000000000000000000, 1.000000000000000000 ) ) ;
#9711=DIRECTION ( 'NONE',  ( 0.000000000000000000, 0.000000000000000000, 1.000000000000000000 ) ) ;
#9722=EDGE_CURVE ( 'NONE', #21448, #1673, #12486, .T. ) ;
#9742=CARTESIAN_POINT ( 'NONE',  ( 0.07874015748031495954, -0.04546065111729338803, -0.4724409448818898127 ) ) ;
#9743=CARTESIAN_POINT ( 'NONE',  ( -0.3031496062992123375, 0.000000000000000000, -0.02362204724409448786 ) ) ;
#9758=ORIENTED_EDGE ( 'NONE', *, *, #9608, .T. ) ;
#9814=CIRCLE ( 'NONE', #8909, 0.2395669291338582696 ) ;
#9824=CARTESIAN_POINT ( 'NONE',  ( -0.07874015748031495954, -0.04546065111729338803, -0.4724409448818898127 ) ) ;
#9829=ORIENTED_EDGE ( 'NONE', *, *, #16589, .F. ) ;
#9845=ORIENTED_EDGE ( 'NONE', *, *, #8377, .T. ) ;
#9847=ADVANCED_FACE ( 'NONE', ( #11061 ), #19991, .F. ) ;
#9886=DIRECTION ( 'NONE',  ( 0.000000000000000000, 0.000000000000000000, 1.000000000000000000 ) ) ;
#9898=EDGE_LOOP ( 'NONE', ( #20575, #24690, #8835, #23811, #19853, #22471, #6532, #25734, #17240, #9327, #19481, #5089, #1339, #22898, #5124, #19598, #25151, #23883, #20480 ) ) ;
#9995=ORIENTED_EDGE ( 'NONE', *, *, #5881, .T. ) ;
#10048=VECTOR ( 'NONE', #18546, 39.37007874015748854 ) ;
#10053=CARTESIAN_POINT ( 'NONE',  ( -0.02916473398703043826, 0.07408303521633090305, -0.4653527282821431355 ) ) ;
#10065=CARTESIAN_POINT ( 'NONE',  ( -1.466875984251968630E-17, 0.000000000000000000, 0.000000000000000000 ) ) ;
#10067=EDGE_CURVE ( 'NONE', #16467, #27805, #22202, .T. ) ;
#10072=CARTESIAN_POINT ( 'NONE',  ( 0.07874015748031489015, 9.642888182262615344E-18, -0.2834645669291338543 ) ) ;
#10090=ORIENTED_EDGE ( 'NONE', *, *, #16372, .T. ) ;
#10120=VECTOR ( 'NONE', #15252, 39.37007874015748854 ) ;
#10127=DIRECTION ( 'NONE',  ( -1.000000000000000000, 0.000000000000000000, 0.000000000000000000 ) ) ;
#10147=DIRECTION ( 'NONE',  ( 0.000000000000000000, 1.000000000000000000, 0.000000000000000000 ) ) ;
#10159=VERTEX_POINT ( 'NONE', #18648 ) ;
#10205=CARTESIAN_POINT ( 'NONE',  ( -0.1181102362204724532, 0.000000000000000000, 0.6228346456772185791 ) ) ;
#10212=CIRCLE ( 'NONE', #24643, 0.08582677165167480748 ) ;
#10215=DIRECTION ( 'NONE',  ( 0.4999999999999998890, 0.8660254037844388186, 0.000000000000000000 ) ) ;
#10218=AXIS2_PLACEMENT_3D ( 'NONE', #24343, #22790, #5123 ) ;
#10225=EDGE_CURVE ( 'NONE', #10260, #20147, #16388, .T. ) ;
#10228=CARTESIAN_POINT ( 'NONE',  ( 0.000000000000000000, 0.000000000000000000, 0.6299212598425196763 ) ) ;
#10260=VERTEX_POINT ( 'NONE', #27707 ) ;
#10266=VERTEX_POINT ( 'NONE', #12713 ) ;
#10319=ADVANCED_FACE ( 'NONE', ( #2463 ), #27189, .T. ) ;
#10345=DIRECTION ( 'NONE',  ( 0.000000000000000000, 0.000000000000000000, -1.000000000000000000 ) ) ;
#10442=DIRECTION ( 'NONE',  ( 0.000000000000000000, 0.000000000000000000, -1.000000000000000000 ) ) ;
#10499=VECTOR ( 'NONE', #26354, 39.37007874015748143 ) ;
#10502=ORIENTED_EDGE ( 'NONE', *, *, #23687, .T. ) ;
#10504=EDGE_LOOP ( 'NONE', ( #12820, #14209, #26077 ) ) ;
#10510=AXIS2_PLACEMENT_3D ( 'NONE', #25965, #4493, #17210 ) ;
#10558=ORIENTED_EDGE ( 'NONE', *, *, #5552, .T. ) ;
#10565=AXIS2_PLACEMENT_3D ( 'NONE', #3126, #11753, #1309 ) ;
#10570=VERTEX_POINT ( 'NONE', #19870 ) ;
#10574=DIRECTION ( 'NONE',  ( -1.000000000000000000, 0.000000000000000000, 0.000000000000000000 ) ) ;
#10586=ORIENTED_EDGE ( 'NONE', *, *, #7177, .F. ) ;
#10602=AXIS2_PLACEMENT_3D ( 'NONE', #12111, #9711, #18593 ) ;
#10609=CARTESIAN_POINT ( 'NONE',  ( 0.07874015748031495954, 0.04546065111729338803, -0.4724409448818898127 ) ) ;
#10622=CARTESIAN_POINT ( 'NONE',  ( -1.928513779527558736E-17, 0.000000000000000000, -0.4448818897637791814 ) ) ;
#10652=LENGTH_MEASURE_WITH_UNIT ( LENGTH_MEASURE( 0.02539999999999999897 ), #25775 ) ;
#10660=ORIENTED_EDGE ( 'NONE', *, *, #21353, .F. ) ;
#10682=ADVANCED_FACE ( 'NONE', ( #15774 ), #13243, .T. ) ;
#10684=LINE ( 'NONE', #19301, #8754 ) ;
#10686=EDGE_CURVE ( 'NONE', #15627, #3542, #20140, .T. ) ;
#10687=ORIENTED_EDGE ( 'NONE', *, *, #5424, .F. ) ;
#10709=CARTESIAN_POINT ( 'NONE',  ( 0.07874015748031495954, 0.04546065111729338803, -0.3779527559055118058 ) ) ;
#10721=CARTESIAN_POINT ( 'NONE',  ( -0.07874015748031495954, -0.03414999754207796723, -0.4724409448818898127 ) ) ;
#10754=DIRECTION ( 'NONE',  ( 0.000000000000000000, 0.000000000000000000, -1.000000000000000000 ) ) ;
#10757=DIRECTION ( 'NONE',  ( -1.000000000000000000, 0.000000000000000000, 0.000000000000000000 ) ) ;
#10770=PLANE ( 'NONE',  #3065 ) ;
#10779=CARTESIAN_POINT ( 'NONE',  ( -0.2395669291338582696, 0.000000000000000000, -0.4566929133858267376 ) ) ;
#10780=ORIENTED_EDGE ( 'NONE', *, *, #16085, .T. ) ;
#10782=DIRECTION ( 'NONE',  ( 0.000000000000000000, -1.000000000000000000, 0.000000000000000000 ) ) ;
#10841=FACE_OUTER_BOUND ( 'NONE', #26254, .T. ) ;
#10846=LINE ( 'NONE', #17740, #179 ) ;
#10862=FACE_OUTER_BOUND ( 'NONE', #20491, .T. ) ;
#10984=ORIENTED_EDGE ( 'NONE', *, *, #18252, .T. ) ;
#11035=AXIS2_PLACEMENT_3D ( 'NONE', #7042, #23875, #17367 ) ;
#11042=EDGE_CURVE ( 'NONE', #27722, #18177, #19522, .T. ) ;
#11043=EDGE_LOOP ( 'NONE', ( #27447, #2457, #23506, #20359 ) ) ;
#11045=ORIENTED_EDGE ( 'NONE', *, *, #1502, .F. ) ;
#11061=FACE_OUTER_BOUND ( 'NONE', #6030, .T. ) ;
#11103=VERTEX_POINT ( 'NONE', #1190 ) ;
#11105=FACE_OUTER_BOUND ( 'NONE', #27290, .T. ) ;
#11130=EDGE_CURVE ( 'NONE', #15627, #12477, #1464, .T. ) ;
#11138=CARTESIAN_POINT ( 'NONE',  ( 0.07874015748031495954, 0.03414999754207796723, -0.4724409448818898127 ) ) ;
#11153=CARTESIAN_POINT ( 'NONE',  ( 0.07874015748031495954, -0.04546065111729338803, -0.4724409448818898127 ) ) ;
#11163=CARTESIAN_POINT ( 'NONE',  ( 0.01935208613492874971, 0.07974837009520491238, -0.4684893292439904489 ) ) ;
#11185=DIRECTION ( 'NONE',  ( -1.000000000000000000, 0.000000000000000000, -0.000000000000000000 ) ) ;
#11186=AXIS2_PLACEMENT_3D ( 'NONE', #15990, #25870, #23759 ) ;
#11203=DIRECTION ( 'NONE',  ( -0.000000000000000000, -0.000000000000000000, -1.000000000000000000 ) ) ;
#11245=CARTESIAN_POINT ( 'NONE',  ( 0.06894484415077314909, -0.05111597790490109150, -0.4724409448818898127 ) ) ;
#11277=DIRECTION ( 'NONE',  ( 0.000000000000000000, 0.000000000000000000, -1.000000000000000000 ) ) ;
#11299=FACE_OUTER_BOUND ( 'NONE', #18934, .T. ) ;
#11321=ORIENTED_EDGE ( 'NONE', *, *, #2768, .T. ) ;
#11323=PLANE ( 'NONE',  #26 ) ;
#11340=DIRECTION ( 'NONE',  ( 0.000000000000000000, 0.000000000000000000, 1.000000000000000000 ) ) ;
#11345=CARTESIAN_POINT ( 'NONE',  ( -4.821283464566928349E-18, 0.000000000000000000, -0.3779527559055118058 ) ) ;
#11392=DIRECTION ( 'NONE',  ( -0.000000000000000000, -0.000000000000000000, -1.000000000000000000 ) ) ;
#11404=DIRECTION ( 'NONE',  ( -1.000000000000000000, 0.000000000000000000, 0.000000000000000000 ) ) ;
#11426=LINE ( 'NONE', #13405, #25714 ) ;
#11454=DIRECTION ( 'NONE',  ( -0.4999999999999998890, -0.8660254037844388186, 0.000000000000000000 ) ) ;
#11467=DIRECTION ( 'NONE',  ( -0.000000000000000000, -0.000000000000000000, -1.000000000000000000 ) ) ;
#11478=ADVANCED_FACE ( 'NONE', ( #13371 ), #17478, .F. ) ;
#11528=VERTEX_POINT ( 'NONE', #26230 ) ;
#11531=ADVANCED_FACE ( 'NONE', ( #4614 ), #27222, .T. ) ;
#11568=EDGE_CURVE ( 'NONE', #5635, #18611, #10846, .T. ) ;
#11574=CARTESIAN_POINT ( 'NONE',  ( 0.06894484415258525511, 0.05111597790624471116, -0.4724409448841456749 ) ) ;
#11588=AXIS2_PLACEMENT_3D ( 'NONE', #5229, #3665, #7923 ) ;
#11599=EDGE_CURVE ( 'NONE', #8441, #8220, #287, .T. ) ;
#11718=DIRECTION ( 'NONE',  ( -1.000000000000000000, 0.000000000000000000, 0.000000000000000000 ) ) ;
#11721=DIRECTION ( 'NONE',  ( 0.000000000000000000, 0.000000000000000000, -1.000000000000000000 ) ) ;
#11726=EDGE_CURVE ( 'NONE', #20809, #1867, #26298, .T. ) ;
#11753=DIRECTION ( 'NONE',  ( -0.000000000000000000, -0.000000000000000000, -1.000000000000000000 ) ) ;
#11760=EDGE_CURVE ( 'NONE', #8441, #2885, #8163, .T. ) ;
#11767=ORIENTED_EDGE ( 'NONE', *, *, #1109, .F. ) ;
#11804=EDGE_LOOP ( 'NONE', ( #25172, #9845, #6829, #7360, #18069, #2227 ) ) ;
#11819=FACE_OUTER_BOUND ( 'NONE', #2407, .T. ) ;
#11825=AXIS2_PLACEMENT_3D ( 'NONE', #12271, #13987, #10147 ) ;
#11828=FACE_OUTER_BOUND ( 'NONE', #14862, .T. ) ;
#11880=ORIENTED_EDGE ( 'NONE', *, *, #7592, .F. ) ;
#11912=CARTESIAN_POINT ( 'NONE',  ( -4.821283464566928349E-18, 0.000000000000000000, -0.3779527559055118058 ) ) ;
#11932=CIRCLE ( 'NONE', #14203, 0.2395669291338582696 ) ;
#11941=DIRECTION ( 'NONE',  ( -1.000000000000000000, 0.000000000000000000, 0.000000000000000000 ) ) ;
#11951=VECTOR ( 'NONE', #19962, 39.37007874015748854 ) ;
#11958=DIRECTION ( 'NONE',  ( -0.000000000000000000, -0.000000000000000000, 1.000000000000000000 ) ) ;
#11988=CARTESIAN_POINT ( 'NONE',  ( 0.000000000000000000, 0.000000000000000000, -0.4724409448818898127 ) ) ;
#11999=LINE ( 'NONE', #21032, #24928 ) ;
#12026=ORIENTED_EDGE ( 'NONE', *, *, #17260, .F. ) ;
#12087=CARTESIAN_POINT ( 'NONE',  ( 0.1110236220424516002, 1.403040230489866364E-17, 0.6299212598425196763 ) ) ;
#12111=CARTESIAN_POINT ( 'NONE',  ( -1.466875984251968630E-17, 0.000000000000000000, -0.4724409448818898127 ) ) ;
#12131=AXIS2_PLACEMENT_3D ( 'NONE', #14237, #22843, #7580 ) ;
#12137=FACE_OUTER_BOUND ( 'NONE', #8092, .T. ) ;
#12157=DIRECTION ( 'NONE',  ( 0.000000000000000000, 0.000000000000000000, -1.000000000000000000 ) ) ;
#12186=ORIENTED_EDGE ( 'NONE', *, *, #14718, .F. ) ;
#12226=ORIENTED_EDGE ( 'NONE', *, *, #11568, .F. ) ;
#12233=DIRECTION ( 'NONE',  ( 0.000000000000000000, 0.000000000000000000, 1.000000000000000000 ) ) ;
#12241=ADVANCED_FACE ( 'NONE', ( #11105 ), #19890, .F. ) ;
#12271=CARTESIAN_POINT ( 'NONE',  ( 0.07874015748031495954, 0.04546065111729338803, -0.4724409448818898127 ) ) ;
#12304=CARTESIAN_POINT ( 'NONE',  ( 0.3031496062992122820, 3.712511950171106268E-17, -0.03543307086614204404 ) ) ;
#12325=DIRECTION ( 'NONE',  ( -1.000000000000000000, 0.000000000000000000, 0.000000000000000000 ) ) ;
#12342=CIRCLE ( 'NONE', #3769, 0.06889763779527552368 ) ;
#12343=ADVANCED_FACE ( 'NONE', ( #791 ), #15417, .F. ) ;
#12358=DIRECTION ( 'NONE',  ( -0.000000000000000000, -0.000000000000000000, -1.000000000000000000 ) ) ;
#12385=AXIS2_PLACEMENT_3D ( 'NONE', #9010, #2653, #19896 ) ;
#12388=CARTESIAN_POINT ( 'NONE',  ( -4.821283464566928349E-18, 0.000000000000000000, -0.3779527559055118058 ) ) ;
#12408=ORIENTED_EDGE ( 'NONE', *, *, #22319, .F. ) ;
#12468=ADVANCED_FACE ( 'NONE', ( #3301 ), #14044, .F. ) ;
#12477=VERTEX_POINT ( 'NONE', #17983 ) ;
#12486=LINE ( 'NONE', #4825, #8252 ) ;
#12510=EDGE_CURVE ( 'NONE', #3579, #4805, #14792, .T. ) ;
#12570=DIRECTION ( 'NONE',  ( -1.000000000000000000, 0.000000000000000000, 0.000000000000000000 ) ) ;
#12601=CARTESIAN_POINT ( 'NONE',  ( 0.02916473398703041744, -0.07408303521633090305, -0.4653527282821430799 ) ) ;
#12615=CARTESIAN_POINT ( 'NONE',  ( -1.928513779527558736E-17, 0.000000000000000000, -0.03543307086614204404 ) ) ;
#12627=DIRECTION ( 'NONE',  ( -1.000000000000000000, 0.000000000000000000, 0.000000000000000000 ) ) ;
#12632=EDGE_CURVE ( 'NONE', #22435, #5635, #26318, .T. ) ;
#12642=CARTESIAN_POINT ( 'NONE',  ( -0.07874015748031495954, 0.04546065111729338803, -0.4724409448818898127 ) ) ;
#12666=MANIFOLD_SOLID_BREP ( 'Cam Follower', #17746 ) ;
#12671=DIMENSIONAL_EXPONENTS ( 1.000000000000000000, 0.000000000000000000, 0.000000000000000000, 0.000000000000000000, 0.000000000000000000, 0.000000000000000000, 0.000000000000000000 ) ;
#12682=ORIENTED_EDGE ( 'NONE', *, *, #25296, .F. ) ;
#12713=CARTESIAN_POINT ( 'NONE',  ( -0.009795313329541911057, -0.08526597544697904485, -0.4724409448818898127 ) ) ;
#12752=ORIENTED_EDGE ( 'NONE', *, *, #14669, .F. ) ;
#12758=PLANE ( 'NONE',  #17225 ) ;
#12770=VERTEX_POINT ( 'NONE', #20098 ) ;
#12781=ORIENTED_EDGE ( 'NONE', *, *, #23168, .T. ) ;
#12820=ORIENTED_EDGE ( 'NONE', *, *, #2360, .F. ) ;
#12830=AXIS2_PLACEMENT_3D ( 'NONE', #15828, #5080, #4950 ) ;
#12835=B_SPLINE_CURVE_WITH_KNOTS ( 'NONE', 3,
 ( #7202, #2944, #11163, #15685, #13288, #572, #5213, #11574 ),
 .UNSPECIFIED., .F., .F.,
 ( 4, 2, 2, 4 ),
 ( 5.336250286839431171E-07, 0.0004434172983718084209, 0.0008863009717149328238, 0.001772068318401181846 ),
 .UNSPECIFIED. ) ;
#12904=B_SPLINE_CURVE_WITH_KNOTS ( 'NONE', 3,
 ( #10721, #21467, #21600, #6488 ),
 .UNSPECIFIED., .F., .F.,
 ( 4, 4 ),
 ( 0.001747226565907129044, 0.002631077521236949331 ),
 .UNSPECIFIED. ) ;
#12911=PRESENTATION_STYLE_ASSIGNMENT (( #21957 ) ) ;
#12936=ORIENTED_EDGE ( 'NONE', *, *, #5472, .T. ) ;
#12959=DIRECTION ( 'NONE',  ( 0.000000000000000000, 0.000000000000000000, -1.000000000000000000 ) ) ;
#12976=CARTESIAN_POINT ( 'NONE',  ( 0.000000000000000000, 0.000000000000000000, -0.4724409448818898127 ) ) ;
#13005=AXIS2_PLACEMENT_3D ( 'NONE', #14939, #12233, #3898 ) ;
#13033=DIRECTION ( 'NONE',  ( 0.000000000000000000, 0.000000000000000000, -1.000000000000000000 ) ) ;
#13070=CARTESIAN_POINT ( 'NONE',  ( -0.07874015748031495954, -0.04546065111729338803, -0.3779527559055118058 ) ) ;
#13079=LINE ( 'NONE', #8428, #4611 ) ;
#13118=FACE_BOUND ( 'NONE', #4727, .T. ) ;
#13124=ORIENTED_EDGE ( 'NONE', *, *, #992, .T. ) ;
#13160=DIRECTION ( 'NONE',  ( -0.8660254037844385966, 0.4999999999999998335, 0.000000000000000000 ) ) ;
#13165=EDGE_CURVE ( 'NONE', #1934, #1673, #13079, .T. ) ;
#13199=CARTESIAN_POINT ( 'NONE',  ( -1.928513779527558736E-17, 0.000000000000000000, -0.03543307086614204404 ) ) ;
#13219=VERTEX_POINT ( 'NONE', #19854 ) ;
#13243=TOROIDAL_SURFACE ( 'NONE', #1072, 0.3031496062992122820, 0.01181102362204755792 ) ;
#13248=ORIENTED_EDGE ( 'NONE', *, *, #11726, .F. ) ;
#13278=ORIENTED_EDGE ( 'NONE', *, *, #8377, .F. ) ;
#13288=CARTESIAN_POINT ( 'NONE',  ( 0.03425350366399289304, 0.07114503267349270299, -0.4653551329966305605 ) ) ;
#13340=ORIENTED_EDGE ( 'NONE', *, *, #1685, .T. ) ;
#13344=FACE_BOUND ( 'NONE', #9898, .T. ) ;
#13370=EDGE_CURVE ( 'NONE', #10570, #12770, #16362, .T. ) ;
#13371=FACE_OUTER_BOUND ( 'NONE', #16982, .T. ) ;
#13388=CARTESIAN_POINT ( 'NONE',  ( -0.03425350366399289304, -0.07114503267349270299, -0.4653551329966305605 ) ) ;
#13397=CARTESIAN_POINT ( 'NONE',  ( 0.000000000000000000, 0.000000000000000000, 0.6299212598425196763 ) ) ;
#13405=CARTESIAN_POINT ( 'NONE',  ( 0.000000000000000000, 0.09092130223458683158, -0.3779527559055118058 ) ) ;
#13471=EDGE_CURVE ( 'NONE', #15836, #5312, #8616, .T. ) ;
#13496=DIRECTION ( 'NONE',  ( -1.000000000000000000, 0.000000000000000000, 0.000000000000000000 ) ) ;
#13507=ADVANCED_FACE ( 'NONE', ( #8371 ), #3684, .T. ) ;
#13513=VECTOR ( 'NONE', #24482, 39.37007874015748143 ) ;
#13519=AXIS2_PLACEMENT_3D ( 'NONE', #17804, #3238, #26426 ) ;
#13524=CARTESIAN_POINT ( 'NONE',  ( 0.000000000000000000, 0.000000000000000000, -0.02362204724409448786 ) ) ;
#13548=DIRECTION ( 'NONE',  ( -1.000000000000000000, 0.000000000000000000, 0.000000000000000000 ) ) ;
#13566=AXIS2_PLACEMENT_3D ( 'NONE', #13629, #16185, #5010 ) ;
#13573=ORIENTED_EDGE ( 'NONE', *, *, #22042, .T. ) ;
#13629=CARTESIAN_POINT ( 'NONE',  ( 0.000000000000000000, 0.000000000000000000, -0.4724409448841456749 ) ) ;
#13646=ORIENTED_EDGE ( 'NONE', *, *, #2466, .T. ) ;
#13689=FACE_OUTER_BOUND ( 'NONE', #23396, .T. ) ;
#13718=ADVANCED_FACE ( 'NONE', ( #12137 ), #859, .F. ) ;
#13732=CARTESIAN_POINT ( 'NONE',  ( -1.466875984251968630E-17, 0.000000000000000000, 0.000000000000000000 ) ) ;
#13784=ORIENTED_EDGE ( 'NONE', *, *, #11760, .F. ) ;
#13857=CARTESIAN_POINT ( 'NONE',  ( 0.000000000000000000, -0.09092130223458683158, -0.4724409448818898127 ) ) ;
#13899=AXIS2_PLACEMENT_3D ( 'NONE', #6941, #10754, #26009 ) ;
#13911=EDGE_CURVE ( 'NONE', #27805, #10159, #18157, .T. ) ;
#13921=DIRECTION ( 'NONE',  ( 0.000000000000000000, 0.000000000000000000, -1.000000000000000000 ) ) ;
#13953=AXIS2_PLACEMENT_3D ( 'NONE', #11988, #23015, #26965 ) ;
#13959=CYLINDRICAL_SURFACE ( 'NONE', #6723, 0.2395669291338582696 ) ;
#13984=EDGE_CURVE ( 'NONE', #12770, #23749, #25885, .T. ) ;
#13987=DIRECTION ( 'NONE',  ( 1.000000000000000000, 0.000000000000000000, 0.000000000000000000 ) ) ;
#13997=CARTESIAN_POINT ( 'NONE',  ( -0.07874015748031495954, 0.04546065111729338803, -0.4724409448818898127 ) ) ;
#13998=CIRCLE ( 'NONE', #2695, 0.06889763779527552368 ) ;
#14015=CARTESIAN_POINT ( 'NONE',  ( 0.06889763779527550980, 8.437527159479786693E-18, -0.3779527559055118058 ) ) ;
#14044=CONICAL_SURFACE ( 'NONE', #14531, 0.08582677165393072516, 0.7853981625000011624 ) ;
#14047=LINE ( 'NONE', #9501, #5130 ) ;
#14075=ORIENTED_EDGE ( 'NONE', *, *, #11042, .F. ) ;
#14084=DIRECTION ( 'NONE',  ( -0.000000000000000000, -0.000000000000000000, -1.000000000000000000 ) ) ;
#14094=CARTESIAN_POINT ( 'NONE',  ( -1.466875984251968630E-17, 0.000000000000000000, -0.4566929133858267376 ) ) ;
#14162=VERTEX_POINT ( 'NONE', #6635 ) ;
#14203=AXIS2_PLACEMENT_3D ( 'NONE', #19630, #26380, #17762 ) ;
#14204=EDGE_LOOP ( 'NONE', ( #17137, #19257, #5915, #22836 ) ) ;
#14209=ORIENTED_EDGE ( 'NONE', *, *, #16694, .T. ) ;
#14210=EDGE_LOOP ( 'NONE', ( #18685, #19394, #25592, #12408 ) ) ;
#14227=DIRECTION ( 'NONE',  ( 1.000000000000000000, 0.000000000000000000, 0.000000000000000000 ) ) ;
#14237=CARTESIAN_POINT ( 'NONE',  ( -4.821283464566928349E-18, 0.000000000000000000, -0.3779527559055118058 ) ) ;
#14250=DIRECTION ( 'NONE',  ( -1.000000000000000000, 0.000000000000000000, 0.000000000000000000 ) ) ;
#14255=ORIENTED_EDGE ( 'NONE', *, *, #2066, .F. ) ;
#14280=CIRCLE ( 'NONE', #18312, 0.3149606299212598381 ) ;
#14295=EDGE_CURVE ( 'NONE', #16467, #7047, #12342, .T. ) ;
#14318=LINE ( 'NONE', #8102, #9273 ) ;
#14341=ORIENTED_EDGE ( 'NONE', *, *, #3995, .T. ) ;
#14370=ORIENTED_EDGE ( 'NONE', *, *, #24231, .T. ) ;
#14417=FACE_OUTER_BOUND ( 'NONE', #4170, .T. ) ;
#14444=CARTESIAN_POINT ( 'NONE',  ( 0.06889763779527550980, 8.437527159479786693E-18, -0.02362204724409468909 ) ) ;
#14465=ORIENTED_EDGE ( 'NONE', *, *, #10225, .F. ) ;
#14495=ADVANCED_FACE ( 'NONE', ( #4834, #895 ), #9203, .T. ) ;
#14531=AXIS2_PLACEMENT_3D ( 'NONE', #26912, #13921, #11941 ) ;
#14539=EDGE_CURVE ( 'NONE', #3868, #27722, #10684, .T. ) ;
#14563=ORIENTED_EDGE ( 'NONE', *, *, #14539, .T. ) ;
#14602=AXIS2_PLACEMENT_3D ( 'NONE', #6475, #12959, #15241 ) ;
#14604=CARTESIAN_POINT ( 'NONE',  ( 0.05938807134538631044, -0.05663358325667527254, -0.4684893292439904489 ) ) ;
#14633=DIRECTION ( 'NONE',  ( 0.000000000000000000, 0.000000000000000000, -1.000000000000000000 ) ) ;
#14669=EDGE_CURVE ( 'NONE', #27454, #18611, #9189, .T. ) ;
#14706=ORIENTED_EDGE ( 'NONE', *, *, #3995, .F. ) ;
#14718=EDGE_CURVE ( 'NONE', #10159, #27805, #23208, .T. ) ;
#14724=AXIS2_PLACEMENT_3D ( 'NONE', #10065, #18671, #8105 ) ;
#14755=CARTESIAN_POINT ( 'NONE',  ( 0.06420467502049351238, -0.05385271582827236975, -0.4702630791244896691 ) ) ;
#14765=AXIS2_PLACEMENT_3D ( 'NONE', #16561, #10345, #27176 ) ;
#14783=CARTESIAN_POINT ( 'NONE',  ( 0.000000000000000000, 0.09092130223458683158, -0.4724409448818898127 ) ) ;
#14787=VECTOR ( 'NONE', #3963, 39.37007874015748143 ) ;
#14792=LINE ( 'NONE', #20695, #19467 ) ;
#14818=ORIENTED_EDGE ( 'NONE', *, *, #12510, .F. ) ;
#14831=( LENGTH_UNIT ( ) NAMED_UNIT ( * ) SI_UNIT ( $, .METRE. ) ) ;
#14862=EDGE_LOOP ( 'NONE', ( #6116, #11767 ) ) ;
#14939=CARTESIAN_POINT ( 'NONE',  ( -1.466875984251968630E-17, 0.000000000000000000, -0.02362204724409448786 ) ) ;
#14952=ADVANCED_FACE ( 'NONE', ( #7208, #23910 ), #2547, .T. ) ;
#15020=ADVANCED_FACE ( 'NONE', ( #7780 ), #18342, .F. ) ;
#15044=DIRECTION ( 'NONE',  ( 0.000000000000000000, 0.000000000000000000, -1.000000000000000000 ) ) ;
#15048=AXIS2_PLACEMENT_3D ( 'NONE', #9242, #20003, #2492 ) ;
#15075=EDGE_CURVE ( 'NONE', #17187, #11528, #27266, .T. ) ;
#15090=DIRECTION ( 'NONE',  ( -1.000000000000000000, 0.000000000000000000, -0.000000000000000000 ) ) ;
#15106=ORIENTED_EDGE ( 'NONE', *, *, #3329, .T. ) ;
#15148=AXIS2_PLACEMENT_3D ( 'NONE', #13524, #22148, #19476 ) ;
#15180=ORIENTED_EDGE ( 'NONE', *, *, #26988, .T. ) ;
#15241=DIRECTION ( 'NONE',  ( -1.000000000000000000, 0.000000000000000000, 0.000000000000000000 ) ) ;
#15252=DIRECTION ( 'NONE',  ( 0.8660254037844385966, -0.4999999999999998335, 0.000000000000000000 ) ) ;
#15254=PRODUCT_DEFINITION_SHAPE ( 'NONE', 'NONE',  #26544 ) ;
#15280=EDGE_CURVE ( 'NONE', #27454, #18611, #24544, .T. ) ;
#15345=ORIENTED_EDGE ( 'NONE', *, *, #14669, .T. ) ;
#15346=CARTESIAN_POINT ( 'NONE',  ( -0.07874015748031495954, -1.062017969535966354E-23, -0.4653543306978102367 ) ) ;
#15357=DIRECTION ( 'NONE',  ( 0.000000000000000000, 0.000000000000000000, -1.000000000000000000 ) ) ;
#15373=ADVANCED_FACE ( 'NONE', ( #173 ), #21745, .F. ) ;
#15402=ADVANCED_FACE ( 'NONE', ( #426, #10862 ), #26381, .F. ) ;
#15413=ADVANCED_FACE ( 'NONE', ( #15665, #13118 ), #24263, .F. ) ;
#15417=CONICAL_SURFACE ( 'NONE', #13566, 0.08582677165393072516, 0.7853981625000011624 ) ;
#15421=ORIENTED_EDGE ( 'NONE', *, *, #19986, .T. ) ;
#15448=ORIENTED_EDGE ( 'NONE', *, *, #20028, .T. ) ;
#15472=CARTESIAN_POINT ( 'NONE',  ( -0.07874015748031495954, 0.02870882010207796015, -0.4702759304817425434 ) ) ;
#15482=CARTESIAN_POINT ( 'NONE',  ( 0.000000000000000000, 0.000000000000000000, -0.3779527559055118058 ) ) ;
#15499=LINE ( 'NONE', #17855, #27756 ) ;
#15515=ORIENTED_EDGE ( 'NONE', *, *, #10225, .T. ) ;
#15574=ORIENTED_EDGE ( 'NONE', *, *, #9288, .F. ) ;
#15578=ORIENTED_EDGE ( 'NONE', *, *, #1109, .T. ) ;
#15579=EDGE_CURVE ( 'NONE', #17370, #4618, #8788, .T. ) ;
#15599=DIRECTION ( 'NONE',  ( 1.000000000000000000, 0.000000000000000000, -0.000000000000000000 ) ) ;
#15608=CARTESIAN_POINT ( 'NONE',  ( -0.07874015748238459567, 0.03414999754297557560, -0.4724409448841456749 ) ) ;
#15618=CARTESIAN_POINT ( 'NONE',  ( -0.2395669291338582696, 0.000000000000000000, -0.4566929133858267376 ) ) ;
#15627=VERTEX_POINT ( 'NONE', #6871 ) ;
#15635=EDGE_LOOP ( 'NONE', ( #22565, #10660, #17402, #19244 ) ) ;
#15663=DIRECTION ( 'NONE',  ( -1.000000000000000000, 0.000000000000000000, 0.000000000000000000 ) ) ;
#15665=FACE_OUTER_BOUND ( 'NONE', #17920, .T. ) ;
#15666=CARTESIAN_POINT ( 'NONE',  ( 0.1181102362204724532, 1.446433227339393765E-17, 0.6299212598425196763 ) ) ;
#15685=CARTESIAN_POINT ( 'NONE',  ( 0.02919171328787628986, 0.07406745870972507306, -0.4660331883676341880 ) ) ;
#15774=FACE_OUTER_BOUND ( 'NONE', #3913, .T. ) ;
#15794=CARTESIAN_POINT ( 'NONE',  ( -0.02919171328787628986, -0.07406745870972507306, -0.4660331883676341880 ) ) ;
#15800=ORIENTED_EDGE ( 'NONE', *, *, #18641, .T. ) ;
#15828=CARTESIAN_POINT ( 'NONE',  ( 0.000000000000000000, 0.000000000000000000, -0.4566929133858267376 ) ) ;
#15836=VERTEX_POINT ( 'NONE', #11245 ) ;
#15898=CONICAL_SURFACE ( 'NONE', #24015, 0.08582677165393072516, 0.7853981625000011624 ) ;
#15908=EDGE_LOOP ( 'NONE', ( #11880, #10558, #21063, #289 ) ) ;
#15968=CARTESIAN_POINT ( 'NONE',  ( -0.3149606299212598381, 0.000000000000000000, -0.03543307086614173179 ) ) ;
#15990=CARTESIAN_POINT ( 'NONE',  ( -1.466875984251968630E-17, 0.000000000000000000, 0.000000000000000000 ) ) ;
#16002=CARTESIAN_POINT ( 'NONE',  ( -0.06420467502049352626, 0.05385271582827238362, -0.4702630791244896691 ) ) ;
#16038=DIRECTION ( 'NONE',  ( 1.000000000000000000, 0.000000000000000000, 0.000000000000000000 ) ) ;
#16057=ORIENTED_EDGE ( 'NONE', *, *, #16884, .F. ) ;
#16085=EDGE_CURVE ( 'NONE', #3868, #7482, #18724, .T. ) ;
#16147=CARTESIAN_POINT ( 'NONE',  ( -0.04448665381632212201, 0.06523692067838750275, -0.4653551329966305605 ) ) ;
#16148=EDGE_CURVE ( 'NONE', #2247, #5635, #26030, .T. ) ;
#16185=DIRECTION ( 'NONE',  ( 0.000000000000000000, 0.000000000000000000, -1.000000000000000000 ) ) ;
#16204=DIRECTION ( 'NONE',  ( -0.000000000000000000, -0.000000000000000000, 1.000000000000000000 ) ) ;
#16231=ORIENTED_EDGE ( 'NONE', *, *, #4506, .T. ) ;
#16271=CARTESIAN_POINT ( 'NONE',  ( 0.000000000000000000, 0.000000000000000000, -0.3779527559055118058 ) ) ;
#16285=EDGE_LOOP ( 'NONE', ( #12936, #27116, #16057, #3597, #16806, #9218, #5083 ) ) ;
#16297=DIRECTION ( 'NONE',  ( 1.000000000000000000, 0.000000000000000000, 0.000000000000000000 ) ) ;
#16334=CIRCLE ( 'NONE', #17246, 0.1181102362204724532 ) ;
#16355=CONICAL_SURFACE ( 'NONE', #1467, 0.1110236220424516002, 0.7853981642948906217 ) ;
#16362=CIRCLE ( 'NONE', #2799, 0.01181102362204758220 ) ;
#16372=EDGE_CURVE ( 'NONE', #11528, #17187, #2686, .T. ) ;
#16388=CIRCLE ( 'NONE', #16804, 0.01181102362204754924 ) ;
#16394=ORIENTED_EDGE ( 'NONE', *, *, #4506, .F. ) ;
#16467=VERTEX_POINT ( 'NONE', #14444 ) ;
#16505=AXIS2_PLACEMENT_3D ( 'NONE', #6252, #2139, #10757 ) ;
#16561=CARTESIAN_POINT ( 'NONE',  ( 0.000000000000000000, 0.000000000000000000, -0.4724409448818898127 ) ) ;
#16589=EDGE_CURVE ( 'NONE', #1934, #147, #19647, .T. ) ;
#16604=EDGE_LOOP ( 'NONE', ( #15578, #9829, #23589, #785, #15574, #23861, #22780 ) ) ;
#16666=ORIENTED_EDGE ( 'NONE', *, *, #3654, .F. ) ;
#16694=EDGE_CURVE ( 'NONE', #24921, #7271, #11426, .T. ) ;
#16721=LINE ( 'NONE', #1884, #24425 ) ;
#16763=CARTESIAN_POINT ( 'NONE',  ( 0.1181102362204724532, 1.446433227339393765E-17, 0.000000000000000000 ) ) ;
#16800=CARTESIAN_POINT ( 'NONE',  ( 0.000000000000000000, 0.000000000000000000, -0.3779527559055118058 ) ) ;
#16804=AXIS2_PLACEMENT_3D ( 'NONE', #12304, #20929, #3834 ) ;
#16806=ORIENTED_EDGE ( 'NONE', *, *, #1685, .F. ) ;
#16868=VECTOR ( 'NONE', #17992, 39.37007874015748854 ) ;
#16879=AXIS2_PLACEMENT_3D ( 'NONE', #9742, #715, #9305 ) ;
#16884=EDGE_CURVE ( 'NONE', #3542, #4805, #8285, .T. ) ;
#16916=AXIS2_PLACEMENT_3D ( 'NONE', #26858, #17456, #19717 ) ;
#16966=DIRECTION ( 'NONE',  ( -0.000000000000000000, -0.000000000000000000, -1.000000000000000000 ) ) ;
#16982=EDGE_LOOP ( 'NONE', ( #20364, #10586, #7361, #24614 ) ) ;
#16985=DIRECTION ( 'NONE',  ( -1.000000000000000000, 0.000000000000000000, -0.000000000000000000 ) ) ;
#17015=CARTESIAN_POINT ( 'NONE',  ( -0.07874015748031495954, -0.03414999754207796723, -0.4724409448818898127 ) ) ;
#17062=CARTESIAN_POINT ( 'NONE',  ( -0.07874015748031495954, -0.04546065111729338803, -0.3779527559055118058 ) ) ;
#17137=ORIENTED_EDGE ( 'NONE', *, *, #26321, .F. ) ;
#17156=DIRECTION ( 'NONE',  ( -1.000000000000000000, -1.224646799147353454E-16, 0.000000000000000000 ) ) ;
#17163=DIRECTION ( 'NONE',  ( -1.000000000000000000, 0.000000000000000000, 0.000000000000000000 ) ) ;
#17187=VERTEX_POINT ( 'NONE', #10072 ) ;
#17210=DIRECTION ( 'NONE',  ( -1.000000000000000000, 0.000000000000000000, 0.000000000000000000 ) ) ;
#17213=ORIENTED_EDGE ( 'NONE', *, *, #9722, .T. ) ;
#17225=AXIS2_PLACEMENT_3D ( 'NONE', #8523, #444, #26138 ) ;
#17240=ORIENTED_EDGE ( 'NONE', *, *, #19523, .T. ) ;
#17246=AXIS2_PLACEMENT_3D ( 'NONE', #17248, #26140, #24018 ) ;
#17248=CARTESIAN_POINT ( 'NONE',  ( 0.000000000000000000, 0.000000000000000000, 0.000000000000000000 ) ) ;
#17260=EDGE_CURVE ( 'NONE', #2756, #20128, #19538, .T. ) ;
#17349=ORIENTED_EDGE ( 'NONE', *, *, #23027, .T. ) ;
#17356=LINE ( 'NONE', #4623, #10120 ) ;
#17365=DIRECTION ( 'NONE',  ( 0.000000000000000000, 0.000000000000000000, -1.000000000000000000 ) ) ;
#17367=DIRECTION ( 'NONE',  ( 1.000000000000000000, 0.000000000000000000, -0.000000000000000000 ) ) ;
#17370=VERTEX_POINT ( 'NONE', #3242 ) ;
#17390=FACE_OUTER_BOUND ( 'NONE', #24275, .T. ) ;
#17402=ORIENTED_EDGE ( 'NONE', *, *, #13370, .T. ) ;
#17404=DIRECTION ( 'NONE',  ( -1.000000000000000000, 0.000000000000000000, 0.000000000000000000 ) ) ;
#17428=( CONVERSION_BASED_UNIT ( 'INCH', #10652 ) LENGTH_UNIT ( ) NAMED_UNIT ( #12671 ) ) ;
#17456=DIRECTION ( 'NONE',  ( -0.000000000000000000, -0.000000000000000000, 1.000000000000000000 ) ) ;
#17478=CYLINDRICAL_SURFACE ( 'NONE', #10510, 0.06889763779527552368 ) ;
#17524=CIRCLE ( 'NONE', #13005, 0.2395669291338582696 ) ;
#17564=CARTESIAN_POINT ( 'NONE',  ( 1.244982677165354375E-18, -0.09092130223458683158, -0.4724409448818898127 ) ) ;
#17576=ORIENTED_EDGE ( 'NONE', *, *, #24370, .F. ) ;
#17586=FACE_OUTER_BOUND ( 'NONE', #19216, .T. ) ;
#17608=ORIENTED_EDGE ( 'NONE', *, *, #8946, .F. ) ;
#17629=CARTESIAN_POINT ( 'NONE',  ( -0.01935208613492874971, -0.07974837009520491238, -0.4684893292439904489 ) ) ;
#17630=CARTESIAN_POINT ( 'NONE',  ( 0.07874015748031495954, 0.01168837908608117392, -0.4660229470383086547 ) ) ;
#17634=DIRECTION ( 'NONE',  ( -0.000000000000000000, -0.000000000000000000, -1.000000000000000000 ) ) ;
#17639=DIRECTION ( 'NONE',  ( -1.000000000000000000, 0.000000000000000000, 0.000000000000000000 ) ) ;
#17669=DIRECTION ( 'NONE',  ( 0.000000000000000000, 0.000000000000000000, -1.000000000000000000 ) ) ;
#17674=( GEOMETRIC_REPRESENTATION_CONTEXT ( 3 ) GLOBAL_UNCERTAINTY_ASSIGNED_CONTEXT ( ( #22888 ) ) GLOBAL_UNIT_ASSIGNED_CONTEXT ( ( #17428, #23937, #8813 ) ) REPRESENTATION_CONTEXT ( 'NONE', 'WORKASPACE' ) ) ;
#17704=CARTESIAN_POINT ( 'NONE',  ( 0.000000000000000000, 0.000000000000000000, 0.000000000000000000 ) ) ;
#17740=CARTESIAN_POINT ( 'NONE',  ( 0.000000000000000000, 0.09092130223458683158, -0.4724409448818898127 ) ) ;
#17746=CLOSED_SHELL ( 'NONE', ( #10682, #20122, #9127, #15373, #3803, #18519, #4835, #5738, #5586, #5357, #8683, #9228, #13507, #20900, #21252, #15413, #9195, #3573, #2381, #13718, #20286, #24044, #9332, #14952, #22863, #19966, #12241, #9847, #12343, #1215, #9167, #12468, #1407, #18809, #14495, #22858, #8150, #15020, #11478, #15402, #6340, #23374, #11531, #10319 ) ) ;
#17762=DIRECTION ( 'NONE',  ( -1.000000000000000000, 0.000000000000000000, 0.000000000000000000 ) ) ;
#17774=CARTESIAN_POINT ( 'NONE',  ( -0.07874015748031495954, 0.04546065111729338803, -0.3779527559055118058 ) ) ;
#17804=CARTESIAN_POINT ( 'NONE',  ( -4.821283464566928349E-18, 0.000000000000000000, -0.2834645669291338543 ) ) ;
#17851=AXIS2_PLACEMENT_3D ( 'NONE', #8383, #25472, #6135 ) ;
#17855=CARTESIAN_POINT ( 'NONE',  ( -0.07874015748031495954, 0.04546065111729338803, -0.3779527559055118058 ) ) ;
#17909=CARTESIAN_POINT ( 'NONE',  ( -0.07874015748031495954, -0.04546065111729338803, -0.4724409448818898127 ) ) ;
#17920=EDGE_LOOP ( 'NONE', ( #17349, #4935 ) ) ;
#17983=CARTESIAN_POINT ( 'NONE',  ( -0.07874015748031489015, 0.000000000000000000, -0.3779527559055118058 ) ) ;
#17992=DIRECTION ( 'NONE',  ( -0.8660254037844382635, 0.5000000000000005551, 0.000000000000000000 ) ) ;
#18023=ORIENTED_EDGE ( 'NONE', *, *, #15579, .F. ) ;
#18028=LINE ( 'NONE', #9156, #24180 ) ;
#18069=ORIENTED_EDGE ( 'NONE', *, *, #11130, .T. ) ;
#18114=CARTESIAN_POINT ( 'NONE',  ( 0.000000000000000000, 0.000000000000000000, 0.6228346456772185791 ) ) ;
#18157=CIRCLE ( 'NONE', #6024, 0.06889763779527552368 ) ;
#18177=VERTEX_POINT ( 'NONE', #22556 ) ;
#18199=CARTESIAN_POINT ( 'NONE',  ( 0.000000000000000000, 0.000000000000000000, -0.4724409448818898127 ) ) ;
#18230=ORIENTED_EDGE ( 'NONE', *, *, #10686, .T. ) ;
#18252=EDGE_CURVE ( 'NONE', #20698, #24921, #3527, .T. ) ;
#18276=ORIENTED_EDGE ( 'NONE', *, *, #27662, .T. ) ;
#18290=CARTESIAN_POINT ( 'NONE',  ( -1.928513779527558736E-17, 0.000000000000000000, -0.4448818897637791814 ) ) ;
#18312=AXIS2_PLACEMENT_3D ( 'NONE', #12615, #25177, #12325 ) ;
#18327=VECTOR ( 'NONE', #15357, 39.37007874015748143 ) ;
#18342=PLANE ( 'NONE',  #25014 ) ;
#18369=ORIENTED_EDGE ( 'NONE', *, *, #26988, .F. ) ;
#18387=DIRECTION ( 'NONE',  ( -0.000000000000000000, -0.000000000000000000, -1.000000000000000000 ) ) ;
#18442=EDGE_CURVE ( 'NONE', #15836, #1934, #2198, .T. ) ;
#18450=VECTOR ( 'NONE', #24105, 39.37007874015748143 ) ;
#18473=PLANE ( 'NONE',  #6877 ) ;
#18483=PLANE ( 'NONE',  #16879 ) ;
#18513=AXIS2_PLACEMENT_3D ( 'NONE', #2744, #19307, #19725 ) ;
#18515=DIRECTION ( 'NONE',  ( 0.000000000000000000, 0.000000000000000000, -1.000000000000000000 ) ) ;
#18519=ADVANCED_FACE ( 'NONE', ( #5054 ), #2525, .T. ) ;
#18546=DIRECTION ( 'NONE',  ( -0.7071067818211350664, 0.000000000000000000, -0.7071067805519599681 ) ) ;
#18590=FACE_OUTER_BOUND ( 'NONE', #9151, .T. ) ;
#18593=DIRECTION ( 'NONE',  ( -1.000000000000000000, 0.000000000000000000, 0.000000000000000000 ) ) ;
#18611=VERTEX_POINT ( 'NONE', #9020 ) ;
#18627=DIRECTION ( 'NONE',  ( -1.000000000000000000, 0.000000000000000000, 0.000000000000000000 ) ) ;
#18629=AXIS2_PLACEMENT_3D ( 'NONE', #4687, #15044, #94 ) ;
#18641=EDGE_CURVE ( 'NONE', #15836, #5312, #889, .T. ) ;
#18648=CARTESIAN_POINT ( 'NONE',  ( -0.06889763779527552368, 0.000000000000000000, -0.2834645669291338543 ) ) ;
#18671=DIRECTION ( 'NONE',  ( 0.000000000000000000, 0.000000000000000000, 1.000000000000000000 ) ) ;
#18675=DIRECTION ( 'NONE',  ( -1.000000000000000000, 0.000000000000000000, 0.000000000000000000 ) ) ;
#18685=ORIENTED_EDGE ( 'NONE', *, *, #14295, .F. ) ;
#18701=DIRECTION ( 'NONE',  ( 0.000000000000000000, -1.000000000000000000, 0.000000000000000000 ) ) ;
#18724=CIRCLE ( 'NONE', #14724, 0.2395669291338582696 ) ;
#18741=CARTESIAN_POINT ( 'NONE',  ( 0.000000000000000000, 0.000000000000000000, -0.4724409448841456749 ) ) ;
#18750=VECTOR ( 'NONE', #7477, 39.37007874015748143 ) ;
#18779=ORIENTED_EDGE ( 'NONE', *, *, #13911, .F. ) ;
#18790=EDGE_CURVE ( 'NONE', #8220, #6378, #340, .T. ) ;
#18809=ADVANCED_FACE ( 'NONE', ( #20107 ), #26596, .T. ) ;
#18829=DIRECTION ( 'NONE',  ( 0.000000000000000000, 0.000000000000000000, -1.000000000000000000 ) ) ;
#18844=CARTESIAN_POINT ( 'NONE',  ( 0.07874015748031495954, 0.04546065111729338803, -0.3779527559055118058 ) ) ;
#18904=CIRCLE ( 'NONE', #1314, 0.1181102362204724532 ) ;
#18909=DIRECTION ( 'NONE',  ( -1.000000000000000000, 0.000000000000000000, 0.000000000000000000 ) ) ;
#18934=EDGE_LOOP ( 'NONE', ( #26567, #26219 ) ) ;
#18981=PLANE ( 'NONE',  #2632 ) ;
#19056=CARTESIAN_POINT ( 'NONE',  ( 0.000000000000000000, 0.000000000000000000, -0.4724409448841456749 ) ) ;
#19196=CARTESIAN_POINT ( 'NONE',  ( -4.821283464566928349E-18, 0.000000000000000000, -0.2834645669291338543 ) ) ;
#19211=CIRCLE ( 'NONE', #16505, 0.07874015748031489015 ) ;
#19216=EDGE_LOOP ( 'NONE', ( #18023, #5430 ) ) ;
#19244=ORIENTED_EDGE ( 'NONE', *, *, #24231, .F. ) ;
#19252=EDGE_LOOP ( 'NONE', ( #14255, #9995, #5273, #7503 ) ) ;
#19257=ORIENTED_EDGE ( 'NONE', *, *, #3329, .F. ) ;
#19293=CARTESIAN_POINT ( 'NONE',  ( 0.2395669291338582696, 2.933848729453403498E-17, 0.000000000000000000 ) ) ;
#19301=CARTESIAN_POINT ( 'NONE',  ( -0.2395669291338582696, 0.000000000000000000, 0.000000000000000000 ) ) ;
#19307=DIRECTION ( 'NONE',  ( 0.000000000000000000, 0.000000000000000000, -1.000000000000000000 ) ) ;
#19315=LENGTH_MEASURE_WITH_UNIT ( LENGTH_MEASURE( 0.02539999999999999897 ), #14831 ) ;
#19375=CARTESIAN_POINT ( 'NONE',  ( 0.000000000000000000, 0.000000000000000000, -0.3779527559055118058 ) ) ;
#19388=FACE_OUTER_BOUND ( 'NONE', #15908, .T. ) ;
#19394=ORIENTED_EDGE ( 'NONE', *, *, #10067, .T. ) ;
#19467=VECTOR ( 'NONE', #18701, 39.37007874015748143 ) ;
#19476=DIRECTION ( 'NONE',  ( 0.000000000000000000, -1.000000000000000000, 0.000000000000000000 ) ) ;
#19481=ORIENTED_EDGE ( 'NONE', *, *, #18641, .F. ) ;
#19495=ORIENTED_EDGE ( 'NONE', *, *, #5071, .T. ) ;
#19522=CIRCLE ( 'NONE', #7330, 0.2395669291338582696 ) ;
#19523=EDGE_CURVE ( 'NONE', #10266, #6015, #1220, .T. ) ;
#19527=EDGE_CURVE ( 'NONE', #20809, #2885, #25212, .T. ) ;
#19538=LINE ( 'NONE', #26429, #9018 ) ;
#19555=DIRECTION ( 'NONE',  ( 0.000000000000000000, 0.000000000000000000, -1.000000000000000000 ) ) ;
#19583=CARTESIAN_POINT ( 'NONE',  ( 0.06894484415506239861, -0.05111597790242464190, -0.4724409448818898127 ) ) ;
#19584=VECTOR ( 'NONE', #23070, 39.37007874015748143 ) ;
#19592=DIRECTION ( 'NONE',  ( 0.8660254037844382635, -0.5000000000000005551, 0.000000000000000000 ) ) ;
#19598=ORIENTED_EDGE ( 'NONE', *, *, #4679, .T. ) ;
#19630=CARTESIAN_POINT ( 'NONE',  ( -1.466875984251968630E-17, 0.000000000000000000, -0.4566929133858267376 ) ) ;
#19647=LINE ( 'NONE', #11153, #19837 ) ;
#19651=CARTESIAN_POINT ( 'NONE',  ( 0.07874015748031495954, 0.03414999754207796723, -0.4724409448818898127 ) ) ;
#19708=DIRECTION ( 'NONE',  ( -1.000000000000000000, 0.000000000000000000, 0.000000000000000000 ) ) ;
#19717=DIRECTION ( 'NONE',  ( -1.000000000000000000, 0.000000000000000000, 0.000000000000000000 ) ) ;
#19725=DIRECTION ( 'NONE',  ( -1.000000000000000000, 0.000000000000000000, 0.000000000000000000 ) ) ;
#19751=EDGE_LOOP ( 'NONE', ( #8179, #16231, #2721 ) ) ;
#19755=CARTESIAN_POINT ( 'NONE',  ( -0.04957542349328453862, -0.06229891813554931657, -0.4653527282821430799 ) ) ;
#19776=FACE_OUTER_BOUND ( 'NONE', #4123, .T. ) ;
#19837=VECTOR ( 'NONE', #8895, 39.37007874015748143 ) ;
#19853=ORIENTED_EDGE ( 'NONE', *, *, #19986, .F. ) ;
#19854=CARTESIAN_POINT ( 'NONE',  ( 0.2395669291338582696, 2.933848729453403498E-17, -0.4566929133858267376 ) ) ;
#19870=CARTESIAN_POINT ( 'NONE',  ( -0.3149606299212598381, 0.000000000000000000, -0.4448818897637791814 ) ) ;
#19878=DIRECTION ( 'NONE',  ( -0.8660254037844383745, -0.5000000000000003331, 0.000000000000000000 ) ) ;
#19890=CONICAL_SURFACE ( 'NONE', #18513, 0.08582677165393072516, 0.7853981625000011624 ) ;
#19895=CARTESIAN_POINT ( 'NONE',  ( 0.07874015748031495954, 0.02306930775746975082, -0.4684758132890252669 ) ) ;
#19896=DIRECTION ( 'NONE',  ( -1.000000000000000000, 0.000000000000000000, 0.000000000000000000 ) ) ;
#19934=CIRCLE ( 'NONE', #122, 0.08582677165167480748 ) ;
#19962=DIRECTION ( 'NONE',  ( -0.8660254037844382635, 0.5000000000000005551, 0.000000000000000000 ) ) ;
#19966=ADVANCED_FACE ( 'NONE', ( #25325 ), #1873, .T. ) ;
#19986=EDGE_CURVE ( 'NONE', #3579, #11103, #26428, .T. ) ;
#19991=CONICAL_SURFACE ( 'NONE', #18629, 0.08582677165393072516, 0.7853981625000011624 ) ;
#20003=DIRECTION ( 'NONE',  ( 0.000000000000000000, 0.000000000000000000, -1.000000000000000000 ) ) ;
#20028=EDGE_CURVE ( 'NONE', #20147, #26096, #14280, .T. ) ;
#20029=CARTESIAN_POINT ( 'NONE',  ( 0.07874015748031495954, -0.02322203878497701435, -0.4680927705512025194 ) ) ;
#20038=DIRECTION ( 'NONE',  ( -0.000000000000000000, -0.000000000000000000, -1.000000000000000000 ) ) ;
#20054=EDGE_CURVE ( 'NONE', #27454, #27801, #14318, .T. ) ;
#20098=CARTESIAN_POINT ( 'NONE',  ( -0.3031496062992123375, 0.000000000000000000, -0.4566929133858267376 ) ) ;
#20107=FACE_OUTER_BOUND ( 'NONE', #26970, .T. ) ;
#20122=ADVANCED_FACE ( 'NONE', ( #19388 ), #4353, .T. ) ;
#20128=VERTEX_POINT ( 'NONE', #6678 ) ;
#20140=LINE ( 'NONE', #9384, #16868 ) ;
#20147=VERTEX_POINT ( 'NONE', #25891 ) ;
#20286=ADVANCED_FACE ( 'NONE', ( #21517 ), #10770, .F. ) ;
#20291=CARTESIAN_POINT ( 'NONE',  ( -0.07874015748031495954, -0.04546065111729338803, -0.3779527559055118058 ) ) ;
#20326=ORIENTED_EDGE ( 'NONE', *, *, #23027, .F. ) ;
#20327=DIRECTION ( 'NONE',  ( 0.8660254037844382635, -0.5000000000000005551, 0.000000000000000000 ) ) ;
#20359=ORIENTED_EDGE ( 'NONE', *, *, #11599, .F. ) ;
#20364=ORIENTED_EDGE ( 'NONE', *, *, #10067, .F. ) ;
#20368=CARTESIAN_POINT ( 'NONE',  ( -0.3031496062992123375, 0.000000000000000000, -0.4448818897637791814 ) ) ;
#20396=EDGE_LOOP ( 'NONE', ( #22547, #1770, #10687, #12026, #16666, #2129, #9235 ) ) ;
#20435=CYLINDRICAL_SURFACE ( 'NONE', #6766, 0.07874015748031489015 ) ;
#20444=ORIENTED_EDGE ( 'NONE', *, *, #241, .F. ) ;
#20474=DIRECTION ( 'NONE',  ( -1.000000000000000000, 0.000000000000000000, -0.000000000000000000 ) ) ;
#20479=AXIS2_PLACEMENT_3D ( 'NONE', #18199, #24432, #22463 ) ;
#20480=ORIENTED_EDGE ( 'NONE', *, *, #11568, .T. ) ;
#20491=EDGE_LOOP ( 'NONE', ( #10090, #8915 ) ) ;
#20519=CARTESIAN_POINT ( 'NONE',  ( -0.04954844419243873560, 0.06231449464215510492, -0.4660331883676340214 ) ) ;
#20573=DIRECTION ( 'NONE',  ( 0.000000000000000000, 0.000000000000000000, -1.000000000000000000 ) ) ;
#20575=ORIENTED_EDGE ( 'NONE', *, *, #15280, .F. ) ;
#20577=DIRECTION ( 'NONE',  ( -1.000000000000000000, 0.000000000000000000, 0.000000000000000000 ) ) ;
#20589=PRODUCT_DEFINITION_FORMATION_WITH_SPECIFIED_SOURCE ( 'ANY', '', #27628, .NOT_KNOWN. ) ;
#20630=ORIENTED_EDGE ( 'NONE', *, *, #23687, .F. ) ;
#20642=EDGE_CURVE ( 'NONE', #21448, #2756, #26522, .T. ) ;
#20695=CARTESIAN_POINT ( 'NONE',  ( -0.07874015748031495954, 0.04546065111729338803, -0.4724409448818898127 ) ) ;
#20698=VERTEX_POINT ( 'NONE', #24007 ) ;
#20809=VERTEX_POINT ( 'NONE', #12087 ) ;
#20900=ADVANCED_FACE ( 'NONE', ( #22094 ), #631, .T. ) ;
#20929=DIRECTION ( 'NONE',  ( -1.224646799147353207E-16, 1.000000000000000000, 0.000000000000000000 ) ) ;
#21032=CARTESIAN_POINT ( 'NONE',  ( 0.07874015748031495954, 0.04546065111729338803, -0.3779527559055118058 ) ) ;
#21063=ORIENTED_EDGE ( 'NONE', *, *, #13984, .F. ) ;
#21068=CARTESIAN_POINT ( 'NONE',  ( 0.04954844419243873560, -0.06231449464215510492, -0.4660331883676339659 ) ) ;
#21080=B_SPLINE_CURVE_WITH_KNOTS ( 'NONE', 3,
 ( #5183, #9554, #17629, #15794, #13388, #19755, #5045, #6909 ),
 .UNSPECIFIED., .F., .F.,
 ( 4, 2, 2, 4 ),
 ( 5.336250286839431171E-07, 0.0004434172983718084209, 0.0008863009717149328238, 0.001772068318401181846 ),
 .UNSPECIFIED. ) ;
#21100=DIRECTION ( 'NONE',  ( -0.000000000000000000, -0.000000000000000000, -1.000000000000000000 ) ) ;
#21248=CARTESIAN_POINT ( 'NONE',  ( -1.466875984251968630E-17, 0.000000000000000000, -0.4566929133858267376 ) ) ;
#21252=ADVANCED_FACE ( 'NONE', ( #2160 ), #11323, .T. ) ;
#21259=ORIENTED_EDGE ( 'NONE', *, *, #26321, .T. ) ;
#21269=DIRECTION ( 'NONE',  ( 0.000000000000000000, 0.000000000000000000, 1.000000000000000000 ) ) ;
#21348=DIRECTION ( 'NONE',  ( -0.000000000000000000, -1.000000000000000000, -0.000000000000000000 ) ) ;
#21353=EDGE_CURVE ( 'NONE', #10570, #23745, #23451, .T. ) ;
#21376=DIRECTION ( 'NONE',  ( -1.000000000000000000, 0.000000000000000000, 0.000000000000000000 ) ) ;
#21389=CARTESIAN_POINT ( 'NONE',  ( -0.06894484415258525511, -0.05111597790624471116, -0.4724409448841456749 ) ) ;
#21390=CIRCLE ( 'NONE', #2436, 0.3031496062992122820 ) ;
#21404=CARTESIAN_POINT ( 'NONE',  ( -4.821283464566928349E-18, 0.000000000000000000, -0.3779527559055118058 ) ) ;
#21409=VERTEX_POINT ( 'NONE', #24442 ) ;
#21448=VERTEX_POINT ( 'NONE', #22910 ) ;
#21467=CARTESIAN_POINT ( 'NONE',  ( -0.07874015748031495954, -0.02322071673952561324, -0.4680922445168273494 ) ) ;
#21517=FACE_OUTER_BOUND ( 'NONE', #16285, .T. ) ;
#21600=CARTESIAN_POINT ( 'NONE',  ( -0.07874015748031495954, -0.01181091161850882261, -0.4653543306978102367 ) ) ;
#21738=CARTESIAN_POINT ( 'NONE',  ( 0.03937007874015749365, 0.06819097667593998491, -0.3779527559055118058 ) ) ;
#21745=CYLINDRICAL_SURFACE ( 'NONE', #12385, 0.07874015748031489015 ) ;
#21773=CARTESIAN_POINT ( 'NONE',  ( -0.07874015748031495954, -0.04546065111729338803, -0.4724409448818898127 ) ) ;
#21829=DIRECTION ( 'NONE',  ( 0.000000000000000000, 0.000000000000000000, -1.000000000000000000 ) ) ;
#21900=AXIS2_PLACEMENT_3D ( 'NONE', #11345, #11203, #2305 ) ;
#21924=ORIENTED_EDGE ( 'NONE', *, *, #4679, .F. ) ;
#21954=AXIS2_PLACEMENT_3D ( 'NONE', #10622, #17669, #17404 ) ;
#21957=SURFACE_STYLE_USAGE ( .BOTH. , #23533 ) ;
#22004=( GEOMETRIC_REPRESENTATION_CONTEXT ( 3 ) GLOBAL_UNCERTAINTY_ASSIGNED_CONTEXT ( ( #5441 ) ) GLOBAL_UNIT_ASSIGNED_CONTEXT ( ( #19, #23301, #25821 ) ) REPRESENTATION_CONTEXT ( 'NONE', 'WORKASPACE' ) ) ;
#22042=EDGE_CURVE ( 'NONE', #11528, #12477, #5589, .T. ) ;
#22046=AXIS2_PLACEMENT_3D ( 'NONE', #15482, #4316, #9090 ) ;
#22048=ORIENTED_EDGE ( 'NONE', *, *, #17260, .T. ) ;
#22051=CONICAL_SURFACE ( 'NONE', #13, 0.08582677165393072516, 0.7853981625000011624 ) ;
#22080=LINE ( 'NONE', #6841, #11951 ) ;
#22094=FACE_OUTER_BOUND ( 'NONE', #9536, .T. ) ;
#22148=DIRECTION ( 'NONE',  ( 0.000000000000000000, 0.000000000000000000, -1.000000000000000000 ) ) ;
#22198=DIRECTION ( 'NONE',  ( -0.000000000000000000, -0.000000000000000000, 1.000000000000000000 ) ) ;
#22202=LINE ( 'NONE', #14015, #8732 ) ;
#22259=DIRECTION ( 'NONE',  ( -1.000000000000000000, 0.000000000000000000, 0.000000000000000000 ) ) ;
#22319=EDGE_CURVE ( 'NONE', #7047, #10159, #6500, .T. ) ;
#22357=CARTESIAN_POINT ( 'NONE',  ( 0.2395669291338582696, 2.933848729453403498E-17, -0.4724409448818898127 ) ) ;
#22388=PRODUCT_CONTEXT ( 'NONE', #9056, 'mechanical' ) ;
#22435=VERTEX_POINT ( 'NONE', #8349 ) ;
#22463=DIRECTION ( 'NONE',  ( -1.000000000000000000, 0.000000000000000000, 0.000000000000000000 ) ) ;
#22465=DIRECTION ( 'NONE',  ( -0.000000000000000000, -0.000000000000000000, -1.000000000000000000 ) ) ;
#22471=ORIENTED_EDGE ( 'NONE', *, *, #12510, .T. ) ;
#22509=DIRECTION ( 'NONE',  ( -1.000000000000000000, 0.000000000000000000, 0.000000000000000000 ) ) ;
#22547=ORIENTED_EDGE ( 'NONE', *, *, #13471, .T. ) ;
#22556=CARTESIAN_POINT ( 'NONE',  ( 0.2395669291338582696, 2.933848729453403498E-17, -0.02362204724409448786 ) ) ;
#22565=ORIENTED_EDGE ( 'NONE', *, *, #5552, .F. ) ;
#22599=FACE_OUTER_BOUND ( 'NONE', #20396, .T. ) ;
#22687=DIRECTION ( 'NONE',  ( 0.000000000000000000, 0.000000000000000000, 1.000000000000000000 ) ) ;
#22698=DIRECTION ( 'NONE',  ( -1.000000000000000000, 0.000000000000000000, 0.000000000000000000 ) ) ;
#22725=AXIS2_PLACEMENT_3D ( 'NONE', #1965, #27260, #10574 ) ;
#22772=LINE ( 'NONE', #5543, #19584 ) ;
#22780=ORIENTED_EDGE ( 'NONE', *, *, #22846, .F. ) ;
#22790=DIRECTION ( 'NONE',  ( -0.000000000000000000, -0.000000000000000000, -1.000000000000000000 ) ) ;
#22797=CARTESIAN_POINT ( 'NONE',  ( 0.000000000000000000, 0.000000000000000000, -0.4724409448818898127 ) ) ;
#22827=ORIENTED_EDGE ( 'NONE', *, *, #27018, .F. ) ;
#22836=ORIENTED_EDGE ( 'NONE', *, *, #15579, .T. ) ;
#22843=DIRECTION ( 'NONE',  ( -0.000000000000000000, -0.000000000000000000, -1.000000000000000000 ) ) ;
#22846=EDGE_CURVE ( 'NONE', #8913, #14162, #4742, .T. ) ;
#22857=DIRECTION ( 'NONE',  ( -1.224646799147353207E-16, 1.000000000000000000, 0.000000000000000000 ) ) ;
#22858=ADVANCED_FACE ( 'NONE', ( #4884 ), #8719, .T. ) ;
#22863=ADVANCED_FACE ( 'NONE', ( #10841 ), #402, .T. ) ;
#22888=UNCERTAINTY_MEASURE_WITH_UNIT (LENGTH_MEASURE( 1.000000000000000082E-05 ), #17428, 'distance_accuracy_value', 'NONE') ;
#22898=ORIENTED_EDGE ( 'NONE', *, *, #617, .F. ) ;
#22910=CARTESIAN_POINT ( 'NONE',  ( 0.07874015748031489015, 0.000000000000000000, -0.3779527559055118058 ) ) ;
#22920=DIRECTION ( 'NONE',  ( -0.000000000000000000, -1.000000000000000000, -0.000000000000000000 ) ) ;
#22934=DIRECTION ( 'NONE',  ( -0.8660254037844383745, -0.5000000000000003331, 0.000000000000000000 ) ) ;
#22957=VECTOR ( 'NONE', #26248, 39.37007874015748143 ) ;
#22977=CIRCLE ( 'NONE', #6302, 0.08582677165167480748 ) ;
#23015=DIRECTION ( 'NONE',  ( 0.000000000000000000, 0.000000000000000000, -1.000000000000000000 ) ) ;
#23024=CARTESIAN_POINT ( 'NONE',  ( -0.06889763779527552368, 0.000000000000000000, -0.02362204724409468909 ) ) ;
#23027=EDGE_CURVE ( 'NONE', #5267, #10260, #7845, .T. ) ;
#23055=PLANE ( 'NONE',  #23995 ) ;
#23058=EDGE_CURVE ( 'NONE', #3542, #12477, #5315, .T. ) ;
#23070=DIRECTION ( 'NONE',  ( -0.7071067805519565264, 0.000000000000000000, -0.7071067818211385081 ) ) ;
#23102=ORIENTED_EDGE ( 'NONE', *, *, #16085, .F. ) ;
#23168=EDGE_CURVE ( 'NONE', #18177, #27722, #17524, .T. ) ;
#23208=CIRCLE ( 'NONE', #10565, 0.06889763779527552368 ) ;
#23210=CARTESIAN_POINT ( 'NONE',  ( -0.07874015748031495954, 0.04546065111729338803, -0.3779527559055118058 ) ) ;
#23301=( NAMED_UNIT ( * ) PLANE_ANGLE_UNIT ( ) SI_UNIT ( $, .RADIAN. ) ) ;
#23324=DIRECTION ( 'NONE',  ( -0.000000000000000000, -0.000000000000000000, -1.000000000000000000 ) ) ;
#23330=CARTESIAN_POINT ( 'NONE',  ( 0.009795313329799274632, -0.08526597544922021044, -0.4724409448841456749 ) ) ;
#23361=CARTESIAN_POINT ( 'NONE',  ( 0.009795313329799274632, -0.08526597544922021044, -0.4724409448841456749 ) ) ;
#23374=ADVANCED_FACE ( 'NONE', ( #17390 ), #26979, .T. ) ;
#23396=EDGE_LOOP ( 'NONE', ( #13248, #841, #13784, #24499 ) ) ;
#23451=CIRCLE ( 'NONE', #23901, 0.3149606299212598381 ) ;
#23462=CARTESIAN_POINT ( 'NONE',  ( 0.3149606299212598381, 3.857155272905049219E-17, -0.4448818897637791814 ) ) ;
#23504=AXIS2_PLACEMENT_3D ( 'NONE', #7156, #20573, #1227 ) ;
#23506=ORIENTED_EDGE ( 'NONE', *, *, #8946, .T. ) ;
#23533=SURFACE_SIDE_STYLE ('',( #6566 ) ) ;
#23572=EDGE_LOOP ( 'NONE', ( #15345, #12226, #7882, #11045, #22827, #19495, #7985 ) ) ;
#23589=ORIENTED_EDGE ( 'NONE', *, *, #13165, .T. ) ;
#23645=DIRECTION ( 'NONE',  ( 0.000000000000000000, 0.000000000000000000, -1.000000000000000000 ) ) ;
#23687=EDGE_CURVE ( 'NONE', #3579, #21409, #12904, .T. ) ;
#23704=AXIS2_PLACEMENT_3D ( 'NONE', #6194, #27802, #15090 ) ;
#23745=VERTEX_POINT ( 'NONE', #23462 ) ;
#23749=VERTEX_POINT ( 'NONE', #4091 ) ;
#23759=DIRECTION ( 'NONE',  ( 1.000000000000000000, 0.000000000000000000, 0.000000000000000000 ) ) ;
#23774=ORIENTED_EDGE ( 'NONE', *, *, #20642, .F. ) ;
#23799=CARTESIAN_POINT ( 'NONE',  ( 0.07874015748031495954, -0.04546065111729338803, -0.3779527559055118058 ) ) ;
#23811=ORIENTED_EDGE ( 'NONE', *, *, #5730, .F. ) ;
#23861=ORIENTED_EDGE ( 'NONE', *, *, #2372, .T. ) ;
#23875=DIRECTION ( 'NONE',  ( 0.000000000000000000, 0.000000000000000000, 1.000000000000000000 ) ) ;
#23883=ORIENTED_EDGE ( 'NONE', *, *, #16148, .T. ) ;
#23901=AXIS2_PLACEMENT_3D ( 'NONE', #597, #22198, #4962 ) ;
#23910=FACE_BOUND ( 'NONE', #4207, .T. ) ;
#23937=( NAMED_UNIT ( * ) PLANE_ANGLE_UNIT ( ) SI_UNIT ( $, .RADIAN. ) ) ;
#23939=CARTESIAN_POINT ( 'NONE',  ( -0.07874015748031495954, 0.005904027120612978866, -0.4653543306978101257 ) ) ;
#23971=DIRECTION ( 'NONE',  ( -0.000000000000000000, -0.000000000000000000, -1.000000000000000000 ) ) ;
#23995=AXIS2_PLACEMENT_3D ( 'NONE', #16271, #12157, #24873 ) ;
#24007=CARTESIAN_POINT ( 'NONE',  ( -0.03937007874015750752, 0.06819097667593998491, -0.3779527559055118058 ) ) ;
#24015=AXIS2_PLACEMENT_3D ( 'NONE', #3645, #1543, #5507 ) ;
#24018=DIRECTION ( 'NONE',  ( 1.000000000000000000, 0.000000000000000000, 0.000000000000000000 ) ) ;
#24042=CARTESIAN_POINT ( 'NONE',  ( 0.07874015748031495954, 0.04546065111729338803, -0.4724409448818898127 ) ) ;
#24044=ADVANCED_FACE ( 'NONE', ( #22599 ), #18483, .F. ) ;
#24045=CARTESIAN_POINT ( 'NONE',  ( 0.000000000000000000, 0.000000000000000000, -0.3779527559055118058 ) ) ;
#24054=LINE ( 'NONE', #26304, #7136 ) ;
#24105=DIRECTION ( 'NONE',  ( 0.000000000000000000, 1.000000000000000000, 0.000000000000000000 ) ) ;
#24116=ORIENTED_EDGE ( 'NONE', *, *, #2570, .T. ) ;
#24158=CARTESIAN_POINT ( 'NONE',  ( -0.07874015748238459567, 0.03414999754297557560, -0.4724409448841456749 ) ) ;
#24180=VECTOR ( 'NONE', #24277, 39.37007874015748143 ) ;
#24231=EDGE_CURVE ( 'NONE', #23749, #12770, #21390, .T. ) ;
#24244=ORIENTED_EDGE ( 'NONE', *, *, #2466, .F. ) ;
#24263=PLANE ( 'NONE',  #15148 ) ;
#24275=EDGE_LOOP ( 'NONE', ( #3699, #294, #9758, #26819 ) ) ;
#24277=DIRECTION ( 'NONE',  ( 0.000000000000000000, 0.000000000000000000, -1.000000000000000000 ) ) ;
#24309=AXIS2_PLACEMENT_3D ( 'NONE', #12388, #1370, #27368 ) ;
#24343=CARTESIAN_POINT ( 'NONE',  ( -1.466875984251968630E-17, 0.000000000000000000, 0.000000000000000000 ) ) ;
#24357=CARTESIAN_POINT ( 'NONE',  ( 0.1181102362204724532, 1.446433227339393765E-17, 0.6228346456772185791 ) ) ;
#24370=EDGE_CURVE ( 'NONE', #27801, #9119, #14047, .T. ) ;
#24386=CIRCLE ( 'NONE', #27130, 0.3149606299212598381 ) ;
#24403=CARTESIAN_POINT ( 'NONE',  ( 0.07874015748031495954, -0.04546065111729338803, -0.4724409448818898127 ) ) ;
#24425=VECTOR ( 'NONE', #21100, 39.37007874015748143 ) ;
#24430=LINE ( 'NONE', #15968, #6285 ) ;
#24432=DIRECTION ( 'NONE',  ( 0.000000000000000000, 0.000000000000000000, -1.000000000000000000 ) ) ;
#24442=CARTESIAN_POINT ( 'NONE',  ( -0.07874015748031495954, -1.062017969535966354E-23, -0.4653543306978102367 ) ) ;
#24482=DIRECTION ( 'NONE',  ( 0.000000000000000000, 0.000000000000000000, -1.000000000000000000 ) ) ;
#24499=ORIENTED_EDGE ( 'NONE', *, *, #9608, .F. ) ;
#24533=CARTESIAN_POINT ( 'NONE',  ( -1.928513779527558736E-17, 0.000000000000000000, -0.03543307086614173179 ) ) ;
#24544=CIRCLE ( 'NONE', #7897, 0.08582677165167480748 ) ;
#24614=ORIENTED_EDGE ( 'NONE', *, *, #14718, .T. ) ;
#24634=ORIENTED_EDGE ( 'NONE', *, *, #2372, .F. ) ;
#24643=AXIS2_PLACEMENT_3D ( 'NONE', #2259, #2130, #18675 ) ;
#24690=ORIENTED_EDGE ( 'NONE', *, *, #20054, .T. ) ;
#24695=CARTESIAN_POINT ( 'NONE',  ( 0.000000000000000000, 0.000000000000000000, 0.6299212598425196763 ) ) ;
#24745=CARTESIAN_POINT ( 'NONE',  ( -0.01928643301569672036, 0.07978627494126659669, -0.4680802598521938696 ) ) ;
#24803=DIRECTION ( 'NONE',  ( -1.000000000000000000, 0.000000000000000000, 0.000000000000000000 ) ) ;
#24847=PLANE ( 'NONE',  #11825 ) ;
#24873=DIRECTION ( 'NONE',  ( -1.000000000000000000, 0.000000000000000000, -0.000000000000000000 ) ) ;
#24889=CARTESIAN_POINT ( 'NONE',  ( -0.05938807134538628962, 0.05663358325667527948, -0.4684893292439903378 ) ) ;
#24900=EDGE_CURVE ( 'NONE', #4805, #9518, #17356, .T. ) ;
#24921=VERTEX_POINT ( 'NONE', #21738 ) ;
#24927=ORIENTED_EDGE ( 'NONE', *, *, #23168, .F. ) ;
#24928=VECTOR ( 'NONE', #1268, 39.37007874015748143 ) ;
#25014=AXIS2_PLACEMENT_3D ( 'NONE', #5517, #9886, #1279 ) ;
#25034=AXIS2_PLACEMENT_3D ( 'NONE', #18741, #3622, #10127 ) ;
#25072=AXIS2_PLACEMENT_3D ( 'NONE', #12642, #25918, #21269 ) ;
#25127=FACE_OUTER_BOUND ( 'NONE', #16604, .T. ) ;
#25151=ORIENTED_EDGE ( 'NONE', *, *, #8524, .F. ) ;
#25172=ORIENTED_EDGE ( 'NONE', *, *, #15075, .F. ) ;
#25177=DIRECTION ( 'NONE',  ( 0.000000000000000000, 0.000000000000000000, -1.000000000000000000 ) ) ;
#25212=LINE ( 'NONE', #4172, #305 ) ;
#25224=VECTOR ( 'NONE', #26011, 39.37007874015748854 ) ;
#25296=EDGE_CURVE ( 'NONE', #10260, #5267, #8790, .T. ) ;
#25302=FACE_OUTER_BOUND ( 'NONE', #19751, .T. ) ;
#25313=DIRECTION ( 'NONE',  ( 0.000000000000000000, 0.000000000000000000, -1.000000000000000000 ) ) ;
#25320=ORIENTED_EDGE ( 'NONE', *, *, #14539, .F. ) ;
#25325=FACE_OUTER_BOUND ( 'NONE', #14204, .T. ) ;
#25355=DIRECTION ( 'NONE',  ( 0.7071067818211350664, 8.659560570126387438E-17, -0.7071067805519599681 ) ) ;
#25378=CYLINDRICAL_SURFACE ( 'NONE', #24309, 0.06889763779527552368 ) ;
#25392=ORIENTED_EDGE ( 'NONE', *, *, #2768, .F. ) ;
#25472=DIRECTION ( 'NONE',  ( 0.000000000000000000, 0.000000000000000000, -1.000000000000000000 ) ) ;
#25523=VECTOR ( 'NONE', #7717, 39.37007874015748854 ) ;
#25528=CIRCLE ( 'NONE', #5689, 0.07874015748031489015 ) ;
#25592=ORIENTED_EDGE ( 'NONE', *, *, #13911, .T. ) ;
#25595=EDGE_LOOP ( 'NONE', ( #15800, #307 ) ) ;
#25647=ORIENTED_EDGE ( 'NONE', *, *, #2360, .T. ) ;
#25674=AXIS2_PLACEMENT_3D ( 'NONE', #13397, #20038, #17639 ) ;
#25714=VECTOR ( 'NONE', #20327, 39.37007874015748854 ) ;
#25734=ORIENTED_EDGE ( 'NONE', *, *, #27574, .F. ) ;
#25748=EDGE_CURVE ( 'NONE', #2247, #3630, #12835, .T. ) ;
#25775=( LENGTH_UNIT ( ) NAMED_UNIT ( * ) SI_UNIT ( $, .METRE. ) ) ;
#25803=DIRECTION ( 'NONE',  ( -0.000000000000000000, -0.000000000000000000, -1.000000000000000000 ) ) ;
#25821=( NAMED_UNIT ( * ) SI_UNIT ( $, .STERADIAN. ) SOLID_ANGLE_UNIT ( ) ) ;
#25858=AXIS2_PLACEMENT_3D ( 'NONE', #6467, #23971, #13496 ) ;
#25863=AXIS2_PLACEMENT_3D ( 'NONE', #17909, #11718, #1139 ) ;
#25870=DIRECTION ( 'NONE',  ( 0.000000000000000000, 0.000000000000000000, 1.000000000000000000 ) ) ;
#25885=CIRCLE ( 'NONE', #22725, 0.3031496062992122820 ) ;
#25891=CARTESIAN_POINT ( 'NONE',  ( 0.3149606299212598381, 3.857155272905049219E-17, -0.03543307086614204404 ) ) ;
#25918=DIRECTION ( 'NONE',  ( -0.4999999999999998890, 0.8660254037844388186, 0.000000000000000000 ) ) ;
#25945=PLANE ( 'NONE',  #23704 ) ;
#25949=VECTOR ( 'NONE', #19592, 39.37007874015748854 ) ;
#25965=CARTESIAN_POINT ( 'NONE',  ( -4.821283464566928349E-18, 0.000000000000000000, -0.3779527559055118058 ) ) ;
#25972=CARTESIAN_POINT ( 'NONE',  ( -4.821283464566928349E-18, 0.000000000000000000, -0.02362204724409468909 ) ) ;
#26009=DIRECTION ( 'NONE',  ( -1.000000000000000000, 0.000000000000000000, 0.000000000000000000 ) ) ;
#26011=DIRECTION ( 'NONE',  ( -0.8660254037844385966, 0.4999999999999998335, 0.000000000000000000 ) ) ;
#26020=CIRCLE ( 'NONE', #771, 0.01181102362204755271 ) ;
#26030=LINE ( 'NONE', #24042, #27781 ) ;
#26076=EDGE_LOOP ( 'NONE', ( #151, #11321, #12781, #25320 ) ) ;
#26077=ORIENTED_EDGE ( 'NONE', *, *, #9288, .T. ) ;
#26096=VERTEX_POINT ( 'NONE', #197 ) ;
#26138=DIRECTION ( 'NONE',  ( 1.000000000000000000, 0.000000000000000000, -0.000000000000000000 ) ) ;
#26140=DIRECTION ( 'NONE',  ( 0.000000000000000000, 0.000000000000000000, 1.000000000000000000 ) ) ;
#26167=DIRECTION ( 'NONE',  ( -0.8660254037844382635, -0.5000000000000005551, 0.000000000000000000 ) ) ;
#26199=DIRECTION ( 'NONE',  ( 0.000000000000000000, -1.000000000000000000, 0.000000000000000000 ) ) ;
#26219=ORIENTED_EDGE ( 'NONE', *, *, #25748, .F. ) ;
#26230=CARTESIAN_POINT ( 'NONE',  ( -0.07874015748031489015, 0.000000000000000000, -0.2834645669291338543 ) ) ;
#26248=DIRECTION ( 'NONE',  ( 0.000000000000000000, 0.000000000000000000, -1.000000000000000000 ) ) ;
#26250=CARTESIAN_POINT ( 'NONE',  ( 0.07874015748031495954, 0.005900511533401469472, -0.4653540093967190039 ) ) ;
#26254=EDGE_LOOP ( 'NONE', ( #18369, #15448, #14341, #534 ) ) ;
#26261=LINE ( 'NONE', #17774, #27807 ) ;
#26298=CIRCLE ( 'NONE', #1956, 0.1110236220424516002 ) ;
#26304=CARTESIAN_POINT ( 'NONE',  ( 0.07874015748031495954, -0.04546065111729338803, -0.3779527559055118058 ) ) ;
#26318=LINE ( 'NONE', #8541, #511 ) ;
#26321=EDGE_CURVE ( 'NONE', #13219, #4618, #5361, .T. ) ;
#26354=DIRECTION ( 'NONE',  ( 0.000000000000000000, 1.000000000000000000, 0.000000000000000000 ) ) ;
#26365=ORIENTED_EDGE ( 'NONE', *, *, #11726, .T. ) ;
#26380=DIRECTION ( 'NONE',  ( 0.000000000000000000, 0.000000000000000000, 1.000000000000000000 ) ) ;
#26381=PLANE ( 'NONE',  #11035 ) ;
#26426=DIRECTION ( 'NONE',  ( -1.000000000000000000, 0.000000000000000000, 0.000000000000000000 ) ) ;
#26428=CIRCLE ( 'NONE', #14765, 0.08582677165167480748 ) ;
#26429=CARTESIAN_POINT ( 'NONE',  ( 0.07874015748031495954, -0.04546065111729338803, -0.3779527559055118058 ) ) ;
#26470=LINE ( 'NONE', #19583, #4061 ) ;
#26485=DIRECTION ( 'NONE',  ( 0.000000000000000000, 0.000000000000000000, -1.000000000000000000 ) ) ;
#26498=AXIS2_PLACEMENT_3D ( 'NONE', #21248, #1465, #12627 ) ;
#26522=CIRCLE ( 'NONE', #2639, 0.07874015748031489015 ) ;
#26544=PRODUCT_DEFINITION ( 'UNKNOWN', '', #20589, #4297 ) ;
#26567=ORIENTED_EDGE ( 'NONE', *, *, #8524, .T. ) ;
#26596=CYLINDRICAL_SURFACE ( 'NONE', #10218, 0.2395669291338582696 ) ;
#26618=DIRECTION ( 'NONE',  ( 0.8660254037844382635, 0.5000000000000005551, 0.000000000000000000 ) ) ;
#26690=CARTESIAN_POINT ( 'NONE',  ( -4.821283464566928349E-18, 0.000000000000000000, -0.2834645669291338543 ) ) ;
#26724=CARTESIAN_POINT ( 'NONE',  ( -0.1110236220424516002, 0.000000000000000000, 0.6299212598425196763 ) ) ;
#26761=DIRECTION ( 'NONE',  ( 0.000000000000000000, 0.000000000000000000, -1.000000000000000000 ) ) ;
#26781=VERTEX_POINT ( 'NONE', #7644 ) ;
#26798=DIRECTION ( 'NONE',  ( -0.000000000000000000, -0.000000000000000000, -1.000000000000000000 ) ) ;
#26819=ORIENTED_EDGE ( 'NONE', *, *, #5881, .F. ) ;
#26858=CARTESIAN_POINT ( 'NONE',  ( -1.928513779527558736E-17, 0.000000000000000000, -0.02362204724409448786 ) ) ;
#26866=LINE ( 'NONE', #23210, #8940 ) ;
#26881=DIRECTION ( 'NONE',  ( 0.000000000000000000, 0.000000000000000000, 1.000000000000000000 ) ) ;
#26912=CARTESIAN_POINT ( 'NONE',  ( 0.000000000000000000, 0.000000000000000000, -0.4724409448841456749 ) ) ;
#26947=CARTESIAN_POINT ( 'NONE',  ( -4.821283464566928349E-18, 0.000000000000000000, -0.02362204724409468909 ) ) ;
#26965=DIRECTION ( 'NONE',  ( -1.000000000000000000, 0.000000000000000000, 0.000000000000000000 ) ) ;
#26970=EDGE_LOOP ( 'NONE', ( #25392, #23102, #14563, #8440 ) ) ;
#26979=CONICAL_SURFACE ( 'NONE', #13899, 0.1110236220424516002, 0.7853981642948906217 ) ;
#26988=EDGE_CURVE ( 'NONE', #20147, #23745, #18028, .T. ) ;
#27018=EDGE_CURVE ( 'NONE', #26781, #20698, #26261, .T. ) ;
#27110=ORIENTED_EDGE ( 'NONE', *, *, #4349, .T. ) ;
#27116=ORIENTED_EDGE ( 'NONE', *, *, #24900, .F. ) ;
#27130=AXIS2_PLACEMENT_3D ( 'NONE', #18290, #16204, #24803 ) ;
#27176=DIRECTION ( 'NONE',  ( -1.000000000000000000, 0.000000000000000000, 0.000000000000000000 ) ) ;
#27189=TOROIDAL_SURFACE ( 'NONE', #8232, 0.3031496062992122820, 0.01181102362204755792 ) ;
#27222=TOROIDAL_SURFACE ( 'NONE', #14602, 0.3031496062992122820, 0.01181102362204755792 ) ;
#27238=VECTOR ( 'NONE', #947, 39.37007874015748143 ) ;
#27253=ORIENTED_EDGE ( 'NONE', *, *, #1444, .T. ) ;
#27260=DIRECTION ( 'NONE',  ( 0.000000000000000000, 0.000000000000000000, -1.000000000000000000 ) ) ;
#27266=CIRCLE ( 'NONE', #6984, 0.07874015748031489015 ) ;
#27290=EDGE_LOOP ( 'NONE', ( #20444, #20630, #15421 ) ) ;
#27368=DIRECTION ( 'NONE',  ( -1.000000000000000000, 0.000000000000000000, 0.000000000000000000 ) ) ;
#27409=EDGE_CURVE ( 'NONE', #8587, #17370, #8690, .T. ) ;
#27447=ORIENTED_EDGE ( 'NONE', *, *, #11760, .T. ) ;
#27454=VERTEX_POINT ( 'NONE', #2997 ) ;
#27562=CARTESIAN_POINT ( 'NONE',  ( -0.06889763779527552368, 0.000000000000000000, -0.3779527559055118058 ) ) ;
#27563=ORIENTED_EDGE ( 'NONE', *, *, #3654, .T. ) ;
#27574=EDGE_CURVE ( 'NONE', #10266, #9518, #10212, .T. ) ;
#27583=LINE ( 'NONE', #10609, #25224 ) ;
#27613=CARTESIAN_POINT ( 'NONE',  ( -0.07874015748031495954, -0.04546065111729338803, -0.3779527559055118058 ) ) ;
#27617=STYLED_ITEM ( 'NONE', ( #12911 ), #12666 ) ;
#27628=PRODUCT ( 'Cam Follower', 'Cam Follower', '', ( #22388 ) ) ;
#27660=CARTESIAN_POINT ( 'NONE',  ( -0.2395669291338582696, 0.000000000000000000, -0.02362204724409448786 ) ) ;
#27662=EDGE_CURVE ( 'NONE', #5267, #26096, #26020, .T. ) ;
#27707=CARTESIAN_POINT ( 'NONE',  ( 0.3031496062992122820, 3.784833611538078052E-17, -0.02362204724409448786 ) ) ;
#27722=VERTEX_POINT ( 'NONE', #27660 ) ;
#27744=EDGE_LOOP ( 'NONE', ( #4949, #18230, #6308 ) ) ;
#27756=VECTOR ( 'NONE', #26618, 39.37007874015748854 ) ;
#27781=VECTOR ( 'NONE', #13160, 39.37007874015748854 ) ;
#27794=VECTOR ( 'NONE', #8679, 39.37007874015748143 ) ;
#27801=VERTEX_POINT ( 'NONE', #13997 ) ;
#27802=DIRECTION ( 'NONE',  ( 0.000000000000000000, 0.000000000000000000, -1.000000000000000000 ) ) ;
#27805=VERTEX_POINT ( 'NONE', #869 ) ;
#27807=VECTOR ( 'NONE', #2387, 39.37007874015748854 ) ;
#27828=AXIS2_PLACEMENT_3D ( 'NONE', #17704, #9217, #2590 ) ;
#27832=CARTESIAN_POINT ( 'NONE',  ( -1.928513779527558736E-17, 0.000000000000000000, -0.03543307086614204404 ) ) ;
#27845=CARTESIAN_POINT ( 'NONE',  ( -4.821283464566928349E-18, 0.000000000000000000, -0.3779527559055118058 ) ) ;
ENDSEC;
END-ISO-10303-21;
